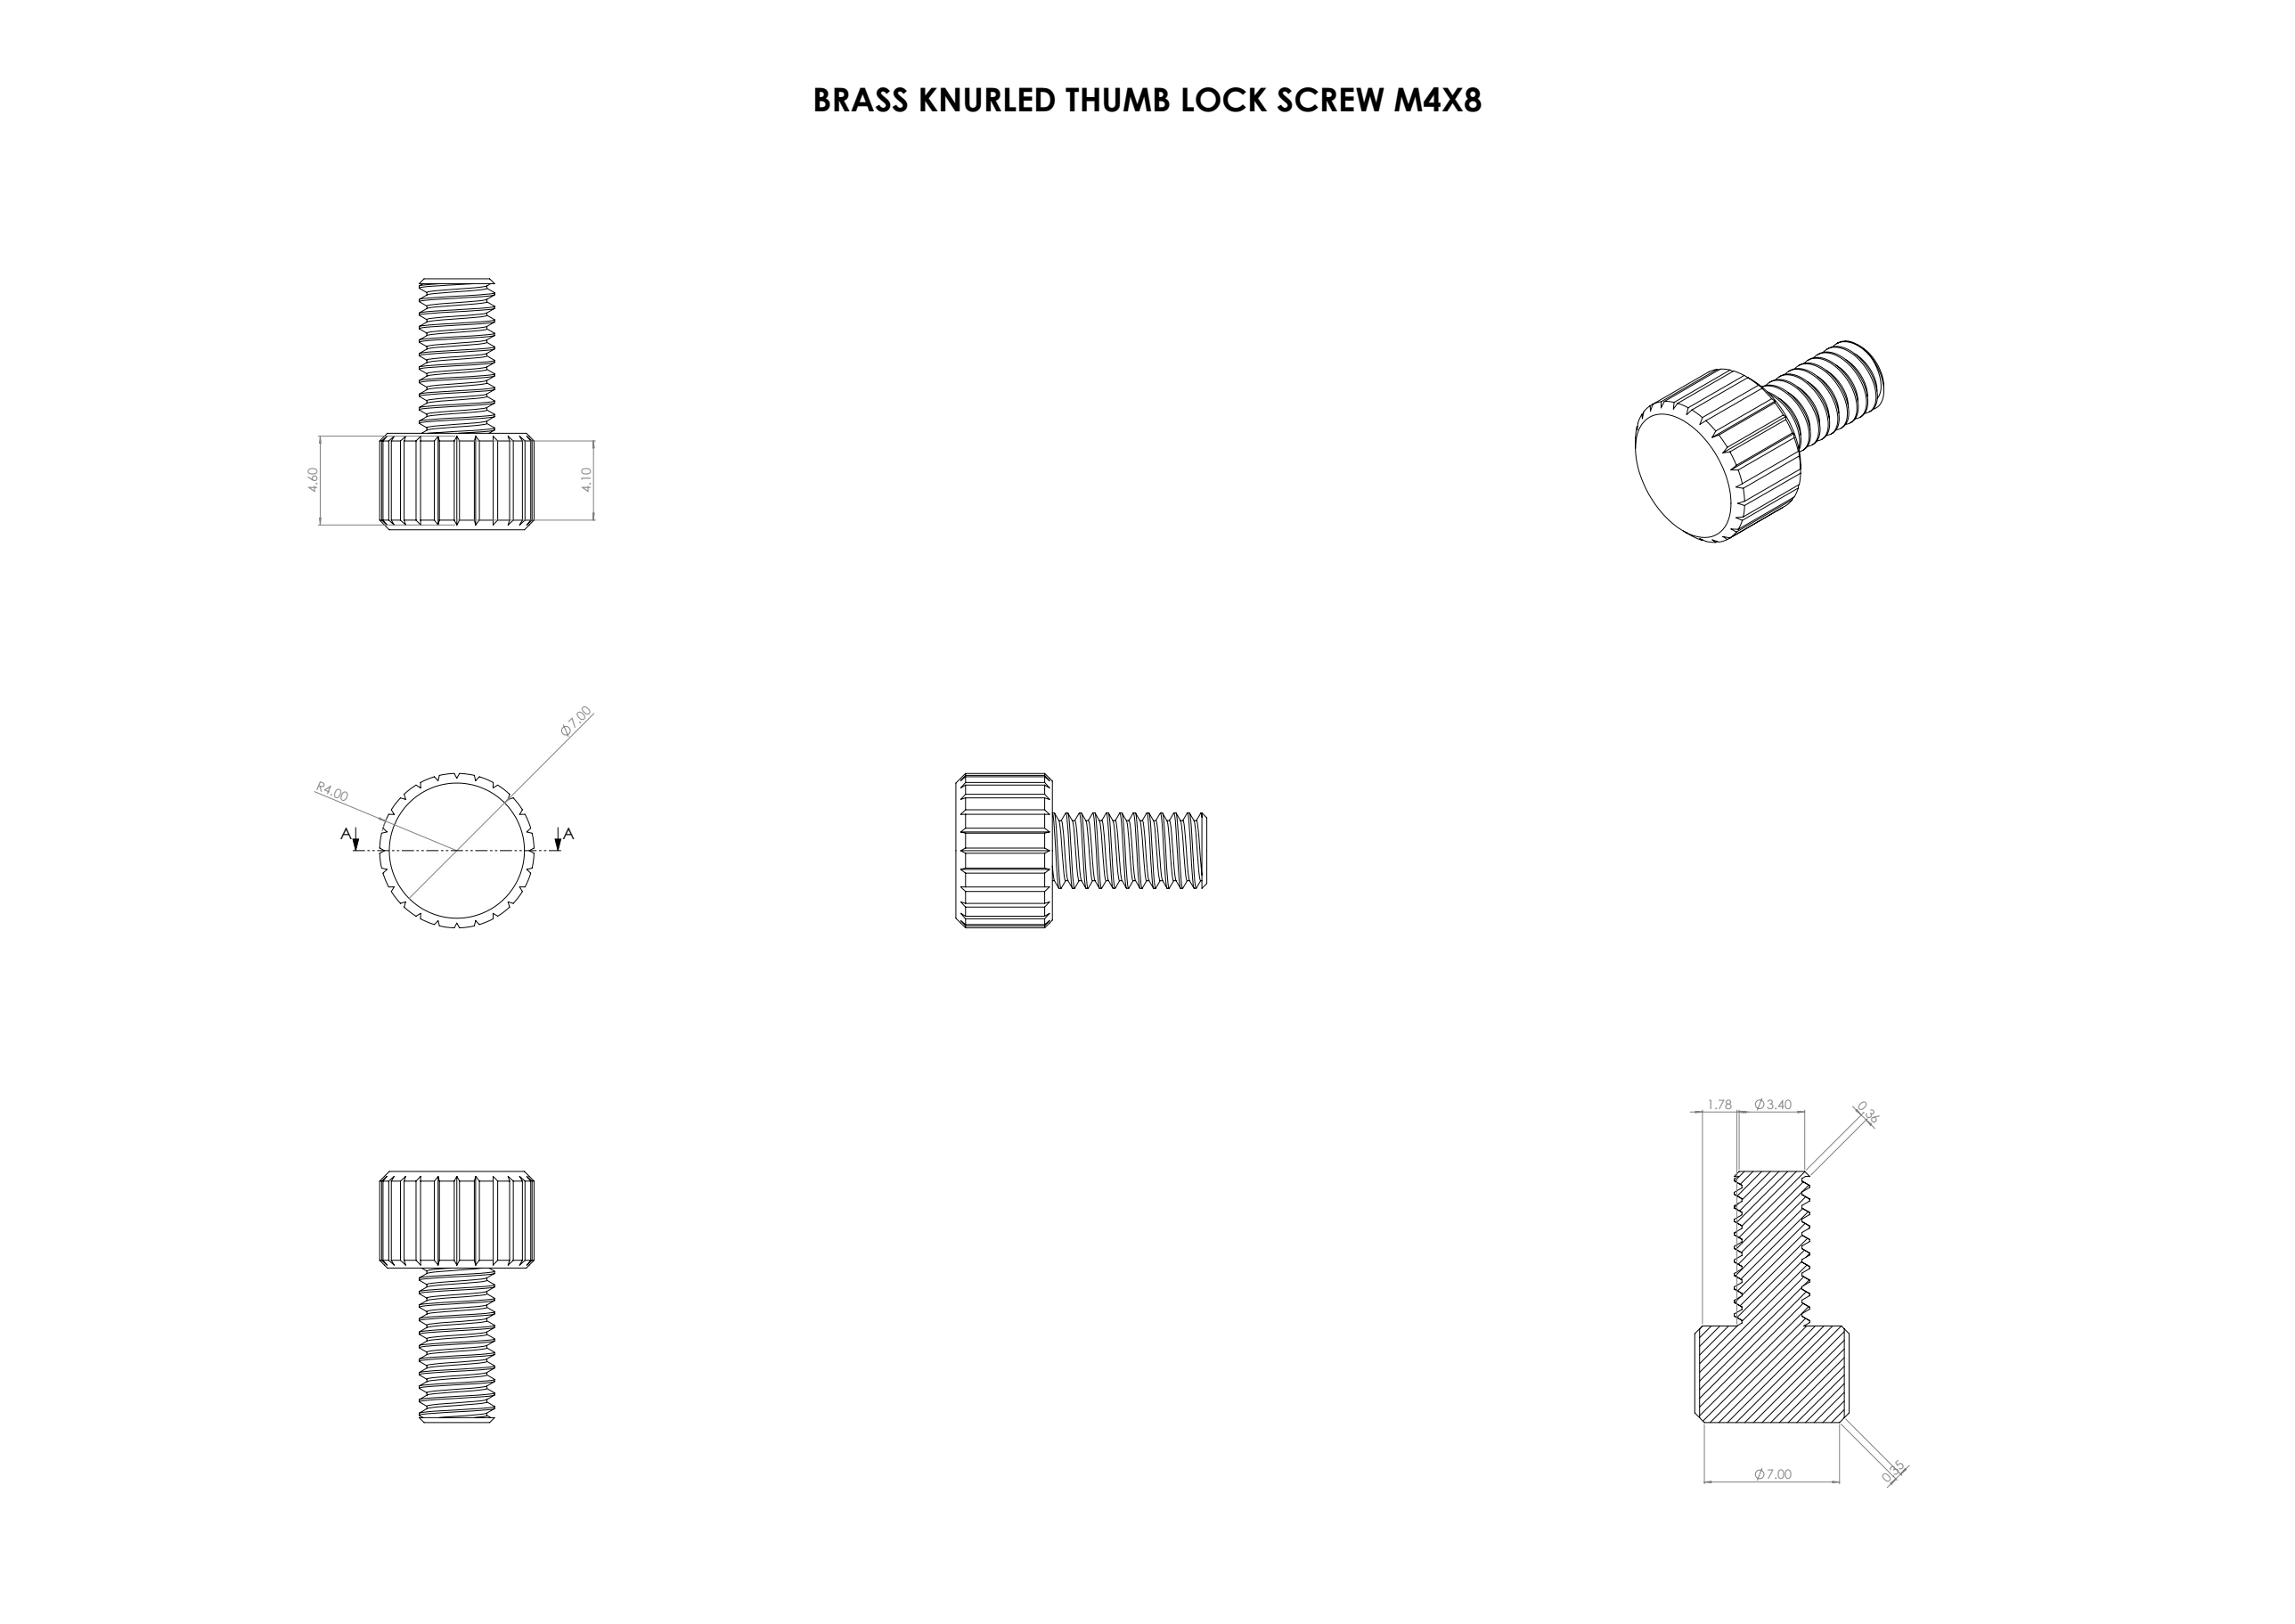
ISO-10303-21;
HEADER;
/* Generated by software containing ST-Developer
 * from STEP Tools, Inc. (www.steptools.com) 
 */

FILE_DESCRIPTION(
/* description */ (''),
/* implementation_level */ '2;1');

FILE_NAME(
/* name */ 
'12_Brass_Knurled_Thumb_Lock_Screw_M4x8.step',
/* time_stamp */ '2026-10-20T10:06:23-07:00',
/* author */ (''),
/* organization */ (''),
/* preprocessor_version */ 'ST-DEVELOPER v20.2',
/* originating_system */ 'Autodesk Translation Framework v15.15.0.0',
/* authorisation */ '');

FILE_SCHEMA (('AUTOMOTIVE_DESIGN { 1 0 10303 214 3 1 1 }'));
ENDSEC;

DATA;
#10=MECHANICAL_DESIGN_GEOMETRIC_PRESENTATION_REPRESENTATION('',(#473),#38611);
#336=(
BOUNDED_CURVE()
B_SPLINE_CURVE(2,(#37921,#37922,#37923),.UNSPECIFIED.,.F.,.F.)
B_SPLINE_CURVE_WITH_KNOTS((3,3),(0.0395243267589975,0.0757709160687003),
 .UNSPECIFIED.)
CURVE()
GEOMETRIC_REPRESENTATION_ITEM()
RATIONAL_B_SPLINE_CURVE((1.00144403367688,1.00138415709391,1.))
REPRESENTATION_ITEM('')
);
#337=(
BOUNDED_CURVE()
B_SPLINE_CURVE(2,(#37927,#37928,#37929),.UNSPECIFIED.,.F.,.F.)
B_SPLINE_CURVE_WITH_KNOTS((3,3),(0.,0.0368264807252771),.UNSPECIFIED.)
CURVE()
GEOMETRIC_REPRESENTATION_ITEM()
RATIONAL_B_SPLINE_CURVE((1.,1.00108727860041,1.00085032920655))
REPRESENTATION_ITEM('')
);
#338=(
BOUNDED_CURVE()
B_SPLINE_CURVE(2,(#37933,#37934,#37935),.UNSPECIFIED.,.F.,.F.)
B_SPLINE_CURVE_WITH_KNOTS((3,3),(0.,0.0362465893096916),.UNSPECIFIED.)
CURVE()
GEOMETRIC_REPRESENTATION_ITEM()
RATIONAL_B_SPLINE_CURVE((1.,1.00138415709372,1.00144403367668))
REPRESENTATION_ITEM('')
);
#339=(
BOUNDED_CURVE()
B_SPLINE_CURVE(2,(#37938,#37939,#37940),.UNSPECIFIED.,.F.,.F.)
B_SPLINE_CURVE_WITH_KNOTS((3,3),(0.023647462726297,0.0604739434515668),
 .UNSPECIFIED.)
CURVE()
GEOMETRIC_REPRESENTATION_ITEM()
RATIONAL_B_SPLINE_CURVE((1.00085032920655,1.0010872786004,1.))
REPRESENTATION_ITEM('')
);
#340=(
BOUNDED_CURVE()
B_SPLINE_CURVE(2,(#37944,#37945,#37946),.UNSPECIFIED.,.F.,.F.)
B_SPLINE_CURVE_WITH_KNOTS((3,3),(0.0395243267590134,0.0757709160687001),
 .UNSPECIFIED.)
CURVE()
GEOMETRIC_REPRESENTATION_ITEM()
RATIONAL_B_SPLINE_CURVE((1.00144403367689,1.00138415709393,1.))
REPRESENTATION_ITEM('')
);
#341=(
BOUNDED_CURVE()
B_SPLINE_CURVE(2,(#37950,#37951,#37952),.UNSPECIFIED.,.F.,.F.)
B_SPLINE_CURVE_WITH_KNOTS((3,3),(0.,0.036826480725251),.UNSPECIFIED.)
CURVE()
GEOMETRIC_REPRESENTATION_ITEM()
RATIONAL_B_SPLINE_CURVE((1.,1.00108727860024,1.00085032920643))
REPRESENTATION_ITEM('')
);
#342=(
BOUNDED_CURVE()
B_SPLINE_CURVE(2,(#37956,#37957,#37958),.UNSPECIFIED.,.F.,.F.)
B_SPLINE_CURVE_WITH_KNOTS((3,3),(0.,0.0362465893097029),.UNSPECIFIED.)
CURVE()
GEOMETRIC_REPRESENTATION_ITEM()
RATIONAL_B_SPLINE_CURVE((1.,1.00138415709418,1.00144403367715))
REPRESENTATION_ITEM('')
);
#343=(
BOUNDED_CURVE()
B_SPLINE_CURVE(2,(#37961,#37962,#37963),.UNSPECIFIED.,.F.,.F.)
B_SPLINE_CURVE_WITH_KNOTS((3,3),(0.0236474627262938,0.060473943451567),
 .UNSPECIFIED.)
CURVE()
GEOMETRIC_REPRESENTATION_ITEM()
RATIONAL_B_SPLINE_CURVE((1.00085032920586,1.00108727859952,1.))
REPRESENTATION_ITEM('')
);
#344=(
BOUNDED_CURVE()
B_SPLINE_CURVE(2,(#37967,#37968,#37969),.UNSPECIFIED.,.F.,.F.)
B_SPLINE_CURVE_WITH_KNOTS((3,3),(0.0395243267590093,0.0757709160687003),
 .UNSPECIFIED.)
CURVE()
GEOMETRIC_REPRESENTATION_ITEM()
RATIONAL_B_SPLINE_CURVE((1.00144403367677,1.00138415709381,1.))
REPRESENTATION_ITEM('')
);
#345=(
BOUNDED_CURVE()
B_SPLINE_CURVE(2,(#37973,#37974,#37975),.UNSPECIFIED.,.F.,.F.)
B_SPLINE_CURVE_WITH_KNOTS((3,3),(0.,0.0368264807252646),.UNSPECIFIED.)
CURVE()
GEOMETRIC_REPRESENTATION_ITEM()
RATIONAL_B_SPLINE_CURVE((1.,1.00108727859976,1.00085032920605))
REPRESENTATION_ITEM('')
);
#346=(
BOUNDED_CURVE()
B_SPLINE_CURVE(2,(#37979,#37980,#37981),.UNSPECIFIED.,.F.,.F.)
B_SPLINE_CURVE_WITH_KNOTS((3,3),(0.,0.0362465893097049),.UNSPECIFIED.)
CURVE()
GEOMETRIC_REPRESENTATION_ITEM()
RATIONAL_B_SPLINE_CURVE((1.,1.0013841570941,1.00144403367707))
REPRESENTATION_ITEM('')
);
#347=(
BOUNDED_CURVE()
B_SPLINE_CURVE(2,(#37984,#37985,#37986),.UNSPECIFIED.,.F.,.F.)
B_SPLINE_CURVE_WITH_KNOTS((3,3),(0.0236474627263067,0.0604739434515669),
 .UNSPECIFIED.)
CURVE()
GEOMETRIC_REPRESENTATION_ITEM()
RATIONAL_B_SPLINE_CURVE((1.00085032920563,1.00108727859922,1.))
REPRESENTATION_ITEM('')
);
#348=(
BOUNDED_CURVE()
B_SPLINE_CURVE(2,(#37990,#37991,#37992),.UNSPECIFIED.,.F.,.F.)
B_SPLINE_CURVE_WITH_KNOTS((3,3),(0.0395243267589975,0.0757709160687003),
 .UNSPECIFIED.)
CURVE()
GEOMETRIC_REPRESENTATION_ITEM()
RATIONAL_B_SPLINE_CURVE((1.00144403367688,1.00138415709391,1.))
REPRESENTATION_ITEM('')
);
#349=(
BOUNDED_CURVE()
B_SPLINE_CURVE(2,(#37996,#37997,#37998),.UNSPECIFIED.,.F.,.F.)
B_SPLINE_CURVE_WITH_KNOTS((3,3),(0.,0.0368264807252771),.UNSPECIFIED.)
CURVE()
GEOMETRIC_REPRESENTATION_ITEM()
RATIONAL_B_SPLINE_CURVE((1.,1.00108727860041,1.00085032920655))
REPRESENTATION_ITEM('')
);
#350=(
BOUNDED_CURVE()
B_SPLINE_CURVE(2,(#38002,#38003,#38004),.UNSPECIFIED.,.F.,.F.)
B_SPLINE_CURVE_WITH_KNOTS((3,3),(0.,0.0362465893096841),.UNSPECIFIED.)
CURVE()
GEOMETRIC_REPRESENTATION_ITEM()
RATIONAL_B_SPLINE_CURVE((1.,1.00138415709402,1.00144403367699))
REPRESENTATION_ITEM('')
);
#351=(
BOUNDED_CURVE()
B_SPLINE_CURVE(2,(#38007,#38008,#38009),.UNSPECIFIED.,.F.,.F.)
B_SPLINE_CURVE_WITH_KNOTS((3,3),(0.0236474627263223,0.0604739434515668),
 .UNSPECIFIED.)
CURVE()
GEOMETRIC_REPRESENTATION_ITEM()
RATIONAL_B_SPLINE_CURVE((1.00085032920605,1.00108727859975,1.))
REPRESENTATION_ITEM('')
);
#352=(
BOUNDED_CURVE()
B_SPLINE_CURVE(2,(#38013,#38014,#38015),.UNSPECIFIED.,.F.,.F.)
B_SPLINE_CURVE_WITH_KNOTS((3,3),(0.0395243267590166,0.0757709160687002),
 .UNSPECIFIED.)
CURVE()
GEOMETRIC_REPRESENTATION_ITEM()
RATIONAL_B_SPLINE_CURVE((1.00144403367685,1.00138415709388,1.))
REPRESENTATION_ITEM('')
);
#353=(
BOUNDED_CURVE()
B_SPLINE_CURVE(2,(#38019,#38020,#38021),.UNSPECIFIED.,.F.,.F.)
B_SPLINE_CURVE_WITH_KNOTS((3,3),(0.,0.0368264807252521),.UNSPECIFIED.)
CURVE()
GEOMETRIC_REPRESENTATION_ITEM()
RATIONAL_B_SPLINE_CURVE((1.,1.00108727859996,1.0008503292062))
REPRESENTATION_ITEM('')
);
#354=(
BOUNDED_CURVE()
B_SPLINE_CURVE(2,(#38025,#38026,#38027),.UNSPECIFIED.,.F.,.F.)
B_SPLINE_CURVE_WITH_KNOTS((3,3),(0.,0.0362465893096854),.UNSPECIFIED.)
CURVE()
GEOMETRIC_REPRESENTATION_ITEM()
RATIONAL_B_SPLINE_CURVE((1.,1.0013841570938,1.00144403367676))
REPRESENTATION_ITEM('')
);
#355=(
BOUNDED_CURVE()
B_SPLINE_CURVE(2,(#38030,#38031,#38032),.UNSPECIFIED.,.F.,.F.)
B_SPLINE_CURVE_WITH_KNOTS((3,3),(0.0236474627263314,0.0604739434515669),
 .UNSPECIFIED.)
CURVE()
GEOMETRIC_REPRESENTATION_ITEM()
RATIONAL_B_SPLINE_CURVE((1.00085032920606,1.00108727859977,1.))
REPRESENTATION_ITEM('')
);
#356=(
BOUNDED_CURVE()
B_SPLINE_CURVE(2,(#38036,#38037,#38038),.UNSPECIFIED.,.F.,.F.)
B_SPLINE_CURVE_WITH_KNOTS((3,3),(0.0395243267589997,0.0757709160687002),
 .UNSPECIFIED.)
CURVE()
GEOMETRIC_REPRESENTATION_ITEM()
RATIONAL_B_SPLINE_CURVE((1.00144403367698,1.00138415709401,1.))
REPRESENTATION_ITEM('')
);
#357=(
BOUNDED_CURVE()
B_SPLINE_CURVE(2,(#38042,#38043,#38044),.UNSPECIFIED.,.F.,.F.)
B_SPLINE_CURVE_WITH_KNOTS((3,3),(0.,0.0368264807252651),.UNSPECIFIED.)
CURVE()
GEOMETRIC_REPRESENTATION_ITEM()
RATIONAL_B_SPLINE_CURVE((1.,1.00108727860044,1.00085032920658))
REPRESENTATION_ITEM('')
);
#358=(
BOUNDED_CURVE()
B_SPLINE_CURVE(2,(#38048,#38049,#38050),.UNSPECIFIED.,.F.,.F.)
B_SPLINE_CURVE_WITH_KNOTS((3,3),(0.,0.0362465893096843),.UNSPECIFIED.)
CURVE()
GEOMETRIC_REPRESENTATION_ITEM()
RATIONAL_B_SPLINE_CURVE((1.,1.00138415709419,1.00144403367717))
REPRESENTATION_ITEM('')
);
#359=(
BOUNDED_CURVE()
B_SPLINE_CURVE(2,(#38053,#38054,#38055),.UNSPECIFIED.,.F.,.F.)
B_SPLINE_CURVE_WITH_KNOTS((3,3),(0.0236474627263023,0.060473943451567),
 .UNSPECIFIED.)
CURVE()
GEOMETRIC_REPRESENTATION_ITEM()
RATIONAL_B_SPLINE_CURVE((1.00085032920674,1.00108727860064,1.))
REPRESENTATION_ITEM('')
);
#360=(
BOUNDED_CURVE()
B_SPLINE_CURVE(2,(#38059,#38060,#38061),.UNSPECIFIED.,.F.,.F.)
B_SPLINE_CURVE_WITH_KNOTS((3,3),(0.0395243267590068,0.0757709160687003),
 .UNSPECIFIED.)
CURVE()
GEOMETRIC_REPRESENTATION_ITEM()
RATIONAL_B_SPLINE_CURVE((1.00144403367694,1.00138415709397,1.))
REPRESENTATION_ITEM('')
);
#361=(
BOUNDED_CURVE()
B_SPLINE_CURVE(2,(#38065,#38066,#38067),.UNSPECIFIED.,.F.,.F.)
B_SPLINE_CURVE_WITH_KNOTS((3,3),(0.,0.0368264807252612),.UNSPECIFIED.)
CURVE()
GEOMETRIC_REPRESENTATION_ITEM()
RATIONAL_B_SPLINE_CURVE((1.,1.00108727859988,1.00085032920614))
REPRESENTATION_ITEM('')
);
#362=(
BOUNDED_CURVE()
B_SPLINE_CURVE(2,(#38071,#38072,#38073),.UNSPECIFIED.,.F.,.F.)
B_SPLINE_CURVE_WITH_KNOTS((3,3),(0.,0.0362465893096925),.UNSPECIFIED.)
CURVE()
GEOMETRIC_REPRESENTATION_ITEM()
RATIONAL_B_SPLINE_CURVE((1.,1.00138415709391,1.00144403367687))
REPRESENTATION_ITEM('')
);
#363=(
BOUNDED_CURVE()
B_SPLINE_CURVE(2,(#38076,#38077,#38078),.UNSPECIFIED.,.F.,.F.)
B_SPLINE_CURVE_WITH_KNOTS((3,3),(0.0236474627263132,0.0604739434515669),
 .UNSPECIFIED.)
CURVE()
GEOMETRIC_REPRESENTATION_ITEM()
RATIONAL_B_SPLINE_CURVE((1.0008503292066,1.00108727860046,1.))
REPRESENTATION_ITEM('')
);
#364=(
BOUNDED_CURVE()
B_SPLINE_CURVE(2,(#38082,#38083,#38084),.UNSPECIFIED.,.F.,.F.)
B_SPLINE_CURVE_WITH_KNOTS((3,3),(0.039524326759018,0.0757709160687002),
 .UNSPECIFIED.)
CURVE()
GEOMETRIC_REPRESENTATION_ITEM()
RATIONAL_B_SPLINE_CURVE((1.00144403367702,1.00138415709405,1.))
REPRESENTATION_ITEM('')
);
#365=(
BOUNDED_CURVE()
B_SPLINE_CURVE(2,(#38088,#38089,#38090),.UNSPECIFIED.,.F.,.F.)
B_SPLINE_CURVE_WITH_KNOTS((3,3),(0.,0.0368264807252612),.UNSPECIFIED.)
CURVE()
GEOMETRIC_REPRESENTATION_ITEM()
RATIONAL_B_SPLINE_CURVE((1.,1.00108727860027,1.00085032920645))
REPRESENTATION_ITEM('')
);
#366=(
BOUNDED_CURVE()
B_SPLINE_CURVE(2,(#38094,#38095,#38096),.UNSPECIFIED.,.F.,.F.)
B_SPLINE_CURVE_WITH_KNOTS((3,3),(0.,0.0362465893096848),.UNSPECIFIED.)
CURVE()
GEOMETRIC_REPRESENTATION_ITEM()
RATIONAL_B_SPLINE_CURVE((1.,1.00138415709428,1.00144403367727))
REPRESENTATION_ITEM('')
);
#367=(
BOUNDED_CURVE()
B_SPLINE_CURVE(2,(#38099,#38100,#38101),.UNSPECIFIED.,.F.,.F.)
B_SPLINE_CURVE_WITH_KNOTS((3,3),(0.0236474627263229,0.060473943451567),
 .UNSPECIFIED.)
CURVE()
GEOMETRIC_REPRESENTATION_ITEM()
RATIONAL_B_SPLINE_CURVE((1.00085032920677,1.00108727860068,1.))
REPRESENTATION_ITEM('')
);
#368=(
BOUNDED_CURVE()
B_SPLINE_CURVE(2,(#38105,#38106,#38107),.UNSPECIFIED.,.F.,.F.)
B_SPLINE_CURVE_WITH_KNOTS((3,3),(0.0395243267590142,0.0757709160687002),
 .UNSPECIFIED.)
CURVE()
GEOMETRIC_REPRESENTATION_ITEM()
RATIONAL_B_SPLINE_CURVE((1.00144403367701,1.00138415709404,1.))
REPRESENTATION_ITEM('')
);
#369=(
BOUNDED_CURVE()
B_SPLINE_CURVE(2,(#38111,#38112,#38113),.UNSPECIFIED.,.F.,.F.)
B_SPLINE_CURVE_WITH_KNOTS((3,3),(0.,0.0368264807252614),.UNSPECIFIED.)
CURVE()
GEOMETRIC_REPRESENTATION_ITEM()
RATIONAL_B_SPLINE_CURVE((1.,1.00108727860056,1.00085032920667))
REPRESENTATION_ITEM('')
);
#370=(
BOUNDED_CURVE()
B_SPLINE_CURVE(2,(#38117,#38118,#38119),.UNSPECIFIED.,.F.,.F.)
B_SPLINE_CURVE_WITH_KNOTS((3,3),(0.,0.0362465893096775),.UNSPECIFIED.)
CURVE()
GEOMETRIC_REPRESENTATION_ITEM()
RATIONAL_B_SPLINE_CURVE((1.,1.00138415709412,1.0014440336771))
REPRESENTATION_ITEM('')
);
#371=(
BOUNDED_CURVE()
B_SPLINE_CURVE(2,(#38122,#38123,#38124),.UNSPECIFIED.,.F.,.F.)
B_SPLINE_CURVE_WITH_KNOTS((3,3),(0.023647462726333,0.060473943451567),
 .UNSPECIFIED.)
CURVE()
GEOMETRIC_REPRESENTATION_ITEM()
RATIONAL_B_SPLINE_CURVE((1.00085032920627,1.00108727860004,1.))
REPRESENTATION_ITEM('')
);
#372=(
BOUNDED_CURVE()
B_SPLINE_CURVE(2,(#38128,#38129,#38130),.UNSPECIFIED.,.F.,.F.)
B_SPLINE_CURVE_WITH_KNOTS((3,3),(0.0395243267590017,0.0757709160687002),
 .UNSPECIFIED.)
CURVE()
GEOMETRIC_REPRESENTATION_ITEM()
RATIONAL_B_SPLINE_CURVE((1.00144403367696,1.00138415709399,1.))
REPRESENTATION_ITEM('')
);
#373=(
BOUNDED_CURVE()
B_SPLINE_CURVE(2,(#38134,#38135,#38136),.UNSPECIFIED.,.F.,.F.)
B_SPLINE_CURVE_WITH_KNOTS((3,3),(0.,0.0368264807252428),.UNSPECIFIED.)
CURVE()
GEOMETRIC_REPRESENTATION_ITEM()
RATIONAL_B_SPLINE_CURVE((1.,1.00108727860007,1.0008503292063))
REPRESENTATION_ITEM('')
);
#374=(
BOUNDED_CURVE()
B_SPLINE_CURVE(2,(#38140,#38141,#38142),.UNSPECIFIED.,.F.,.F.)
B_SPLINE_CURVE_WITH_KNOTS((3,3),(0.,0.036246589309685),.UNSPECIFIED.)
CURVE()
GEOMETRIC_REPRESENTATION_ITEM()
RATIONAL_B_SPLINE_CURVE((1.,1.00138415709379,1.00144403367676))
REPRESENTATION_ITEM('')
);
#375=(
BOUNDED_CURVE()
B_SPLINE_CURVE(2,(#38145,#38146,#38147),.UNSPECIFIED.,.F.,.F.)
B_SPLINE_CURVE_WITH_KNOTS((3,3),(0.0236474627262961,0.060473943451567),
 .UNSPECIFIED.)
CURVE()
GEOMETRIC_REPRESENTATION_ITEM()
RATIONAL_B_SPLINE_CURVE((1.00085032920624,1.0010872786,1.))
REPRESENTATION_ITEM('')
);
#376=(
BOUNDED_CURVE()
B_SPLINE_CURVE(2,(#38151,#38152,#38153),.UNSPECIFIED.,.F.,.F.)
B_SPLINE_CURVE_WITH_KNOTS((3,3),(0.0395243267590158,0.0757709160687002),
 .UNSPECIFIED.)
CURVE()
GEOMETRIC_REPRESENTATION_ITEM()
RATIONAL_B_SPLINE_CURVE((1.0014440336769,1.00138415709393,1.))
REPRESENTATION_ITEM('')
);
#377=(
BOUNDED_CURVE()
B_SPLINE_CURVE(2,(#38157,#38158,#38159),.UNSPECIFIED.,.F.,.F.)
B_SPLINE_CURVE_WITH_KNOTS((3,3),(0.,0.0368264807252534),.UNSPECIFIED.)
CURVE()
GEOMETRIC_REPRESENTATION_ITEM()
RATIONAL_B_SPLINE_CURVE((1.,1.00108727860033,1.00085032920649))
REPRESENTATION_ITEM('')
);
#378=(
BOUNDED_CURVE()
B_SPLINE_CURVE(2,(#38163,#38164,#38165),.UNSPECIFIED.,.F.,.F.)
B_SPLINE_CURVE_WITH_KNOTS((3,3),(0.,0.0362465893096853),.UNSPECIFIED.)
CURVE()
GEOMETRIC_REPRESENTATION_ITEM()
RATIONAL_B_SPLINE_CURVE((1.,1.00138415709412,1.0014440336771))
REPRESENTATION_ITEM('')
);
#379=(
BOUNDED_CURVE()
B_SPLINE_CURVE(2,(#38168,#38169,#38170),.UNSPECIFIED.,.F.,.F.)
B_SPLINE_CURVE_WITH_KNOTS((3,3),(0.0236474627263147,0.060473943451567),
 .UNSPECIFIED.)
CURVE()
GEOMETRIC_REPRESENTATION_ITEM()
RATIONAL_B_SPLINE_CURVE((1.00085032920646,1.00108727860028,1.))
REPRESENTATION_ITEM('')
);
#380=(
BOUNDED_CURVE()
B_SPLINE_CURVE(2,(#38174,#38175,#38176),.UNSPECIFIED.,.F.,.F.)
B_SPLINE_CURVE_WITH_KNOTS((3,3),(0.0395243267590156,0.0757709160687002),
 .UNSPECIFIED.)
CURVE()
GEOMETRIC_REPRESENTATION_ITEM()
RATIONAL_B_SPLINE_CURVE((1.00144403367684,1.00138415709387,1.))
REPRESENTATION_ITEM('')
);
#381=(
BOUNDED_CURVE()
B_SPLINE_CURVE(2,(#38180,#38181,#38182),.UNSPECIFIED.,.F.,.F.)
B_SPLINE_CURVE_WITH_KNOTS((3,3),(0.,0.0368264807252693),.UNSPECIFIED.)
CURVE()
GEOMETRIC_REPRESENTATION_ITEM()
RATIONAL_B_SPLINE_CURVE((1.,1.00108727859986,1.00085032920613))
REPRESENTATION_ITEM('')
);
#382=(
BOUNDED_CURVE()
B_SPLINE_CURVE(2,(#38186,#38187,#38188),.UNSPECIFIED.,.F.,.F.)
B_SPLINE_CURVE_WITH_KNOTS((3,3),(0.,0.0362465893096901),.UNSPECIFIED.)
CURVE()
GEOMETRIC_REPRESENTATION_ITEM()
RATIONAL_B_SPLINE_CURVE((1.,1.00138415709395,1.00144403367692))
REPRESENTATION_ITEM('')
);
#383=(
BOUNDED_CURVE()
B_SPLINE_CURVE(2,(#38191,#38192,#38193),.UNSPECIFIED.,.F.,.F.)
B_SPLINE_CURVE_WITH_KNOTS((3,3),(0.0236474627263255,0.0604739434515669),
 .UNSPECIFIED.)
CURVE()
GEOMETRIC_REPRESENTATION_ITEM()
RATIONAL_B_SPLINE_CURVE((1.0008503292064,1.00108727860021,1.))
REPRESENTATION_ITEM('')
);
#384=(
BOUNDED_CURVE()
B_SPLINE_CURVE(2,(#38197,#38198,#38199),.UNSPECIFIED.,.F.,.F.)
B_SPLINE_CURVE_WITH_KNOTS((3,3),(0.0395243267590232,0.0757709160687003),
 .UNSPECIFIED.)
CURVE()
GEOMETRIC_REPRESENTATION_ITEM()
RATIONAL_B_SPLINE_CURVE((1.0014440336771,1.00138415709412,1.))
REPRESENTATION_ITEM('')
);
#385=(
BOUNDED_CURVE()
B_SPLINE_CURVE(2,(#38203,#38204,#38205),.UNSPECIFIED.,.F.,.F.)
B_SPLINE_CURVE_WITH_KNOTS((3,3),(0.,0.0368264807252497),.UNSPECIFIED.)
CURVE()
GEOMETRIC_REPRESENTATION_ITEM()
RATIONAL_B_SPLINE_CURVE((1.,1.00108727859942,1.00085032920579))
REPRESENTATION_ITEM('')
);
#386=(
BOUNDED_CURVE()
B_SPLINE_CURVE(2,(#38209,#38210,#38211),.UNSPECIFIED.,.F.,.F.)
B_SPLINE_CURVE_WITH_KNOTS((3,3),(0.,0.0362465893096849),.UNSPECIFIED.)
CURVE()
GEOMETRIC_REPRESENTATION_ITEM()
RATIONAL_B_SPLINE_CURVE((1.,1.00138415709363,1.00144403367659))
REPRESENTATION_ITEM('')
);
#387=(
BOUNDED_CURVE()
B_SPLINE_CURVE(2,(#38214,#38215,#38216),.UNSPECIFIED.,.F.,.F.)
B_SPLINE_CURVE_WITH_KNOTS((3,3),(0.0236474627263162,0.060473943451567),
 .UNSPECIFIED.)
CURVE()
GEOMETRIC_REPRESENTATION_ITEM()
RATIONAL_B_SPLINE_CURVE((1.00085032920633,1.00108727860012,1.))
REPRESENTATION_ITEM('')
);
#388=(
BOUNDED_CURVE()
B_SPLINE_CURVE(2,(#38220,#38221,#38222),.UNSPECIFIED.,.F.,.F.)
B_SPLINE_CURVE_WITH_KNOTS((3,3),(0.0395243267590082,0.0757709160687002),
 .UNSPECIFIED.)
CURVE()
GEOMETRIC_REPRESENTATION_ITEM()
RATIONAL_B_SPLINE_CURVE((1.00144403367716,1.00138415709418,1.))
REPRESENTATION_ITEM('')
);
#389=(
BOUNDED_CURVE()
B_SPLINE_CURVE(2,(#38226,#38227,#38228),.UNSPECIFIED.,.F.,.F.)
B_SPLINE_CURVE_WITH_KNOTS((3,3),(0.,0.0368264807252609),.UNSPECIFIED.)
CURVE()
GEOMETRIC_REPRESENTATION_ITEM()
RATIONAL_B_SPLINE_CURVE((1.,1.00108727859987,1.00085032920614))
REPRESENTATION_ITEM('')
);
#390=(
BOUNDED_CURVE()
B_SPLINE_CURVE(2,(#38232,#38233,#38234),.UNSPECIFIED.,.F.,.F.)
B_SPLINE_CURVE_WITH_KNOTS((3,3),(0.,0.0362465893096812),.UNSPECIFIED.)
CURVE()
GEOMETRIC_REPRESENTATION_ITEM()
RATIONAL_B_SPLINE_CURVE((1.,1.0013841570937,1.00144403367666))
REPRESENTATION_ITEM('')
);
#391=(
BOUNDED_CURVE()
B_SPLINE_CURVE(2,(#38237,#38238,#38239),.UNSPECIFIED.,.F.,.F.)
B_SPLINE_CURVE_WITH_KNOTS((3,3),(0.0236474627263107,0.0604739434515669),
 .UNSPECIFIED.)
CURVE()
GEOMETRIC_REPRESENTATION_ITEM()
RATIONAL_B_SPLINE_CURVE((1.00085032920669,1.00108727860058,1.))
REPRESENTATION_ITEM('')
);
#392=(
BOUNDED_CURVE()
B_SPLINE_CURVE(2,(#38243,#38244,#38245),.UNSPECIFIED.,.F.,.F.)
B_SPLINE_CURVE_WITH_KNOTS((3,3),(0.0395243267589996,0.0757709160687002),
 .UNSPECIFIED.)
CURVE()
GEOMETRIC_REPRESENTATION_ITEM()
RATIONAL_B_SPLINE_CURVE((1.00144403367705,1.00138415709408,1.))
REPRESENTATION_ITEM('')
);
#393=(
BOUNDED_CURVE()
B_SPLINE_CURVE(2,(#38249,#38250,#38251),.UNSPECIFIED.,.F.,.F.)
B_SPLINE_CURVE_WITH_KNOTS((3,3),(0.,0.0368264807252541),.UNSPECIFIED.)
CURVE()
GEOMETRIC_REPRESENTATION_ITEM()
RATIONAL_B_SPLINE_CURVE((1.,1.00108727860017,1.00085032920637))
REPRESENTATION_ITEM('')
);
#394=(
BOUNDED_CURVE()
B_SPLINE_CURVE(2,(#38255,#38256,#38257),.UNSPECIFIED.,.F.,.F.)
B_SPLINE_CURVE_WITH_KNOTS((3,3),(0.,0.0362465893096801),.UNSPECIFIED.)
CURVE()
GEOMETRIC_REPRESENTATION_ITEM()
RATIONAL_B_SPLINE_CURVE((1.,1.00138415709414,1.00144403367712))
REPRESENTATION_ITEM('')
);
#395=(
BOUNDED_CURVE()
B_SPLINE_CURVE(2,(#38260,#38261,#38262),.UNSPECIFIED.,.F.,.F.)
B_SPLINE_CURVE_WITH_KNOTS((3,3),(0.0236474627263037,0.060473943451567),
 .UNSPECIFIED.)
CURVE()
GEOMETRIC_REPRESENTATION_ITEM()
RATIONAL_B_SPLINE_CURVE((1.00085032920654,1.00108727860038,1.))
REPRESENTATION_ITEM('')
);
#396=(
BOUNDED_CURVE()
B_SPLINE_CURVE(2,(#38266,#38267,#38268),.UNSPECIFIED.,.F.,.F.)
B_SPLINE_CURVE_WITH_KNOTS((3,3),(0.0395243267590246,0.0757709160687002),
 .UNSPECIFIED.)
CURVE()
GEOMETRIC_REPRESENTATION_ITEM()
RATIONAL_B_SPLINE_CURVE((1.00144403367709,1.00138415709411,1.))
REPRESENTATION_ITEM('')
);
#397=(
BOUNDED_CURVE()
B_SPLINE_CURVE(2,(#38272,#38273,#38274),.UNSPECIFIED.,.F.,.F.)
B_SPLINE_CURVE_WITH_KNOTS((3,3),(0.,0.0368264807252722),.UNSPECIFIED.)
CURVE()
GEOMETRIC_REPRESENTATION_ITEM()
RATIONAL_B_SPLINE_CURVE((1.,1.00108727859999,1.00085032920623))
REPRESENTATION_ITEM('')
);
#398=(
BOUNDED_CURVE()
B_SPLINE_CURVE(2,(#38278,#38279,#38280),.UNSPECIFIED.,.F.,.F.)
B_SPLINE_CURVE_WITH_KNOTS((3,3),(0.,0.036246589309683),.UNSPECIFIED.)
CURVE()
GEOMETRIC_REPRESENTATION_ITEM()
RATIONAL_B_SPLINE_CURVE((1.,1.00138415709414,1.00144403367712))
REPRESENTATION_ITEM('')
);
#399=(
BOUNDED_CURVE()
B_SPLINE_CURVE(2,(#38283,#38284,#38285),.UNSPECIFIED.,.F.,.F.)
B_SPLINE_CURVE_WITH_KNOTS((3,3),(0.0236474627263149,0.060473943451567),
 .UNSPECIFIED.)
CURVE()
GEOMETRIC_REPRESENTATION_ITEM()
RATIONAL_B_SPLINE_CURVE((1.00085032920643,1.00108727860025,1.))
REPRESENTATION_ITEM('')
);
#400=(
BOUNDED_CURVE()
B_SPLINE_CURVE(2,(#38289,#38290,#38291),.UNSPECIFIED.,.F.,.F.)
B_SPLINE_CURVE_WITH_KNOTS((3,3),(0.0395243267590166,0.0757709160687002),
 .UNSPECIFIED.)
CURVE()
GEOMETRIC_REPRESENTATION_ITEM()
RATIONAL_B_SPLINE_CURVE((1.00144403367727,1.00138415709429,1.))
REPRESENTATION_ITEM('')
);
#401=(
BOUNDED_CURVE()
B_SPLINE_CURVE(2,(#38295,#38296,#38297),.UNSPECIFIED.,.F.,.F.)
B_SPLINE_CURVE_WITH_KNOTS((3,3),(0.,0.0368264807252481),.UNSPECIFIED.)
CURVE()
GEOMETRIC_REPRESENTATION_ITEM()
RATIONAL_B_SPLINE_CURVE((1.,1.00108727859946,1.00085032920581))
REPRESENTATION_ITEM('')
);
#402=(
BOUNDED_CURVE()
B_SPLINE_CURVE(2,(#38301,#38302,#38303),.UNSPECIFIED.,.F.,.F.)
B_SPLINE_CURVE_WITH_KNOTS((3,3),(0.,0.0362465893096797),.UNSPECIFIED.)
CURVE()
GEOMETRIC_REPRESENTATION_ITEM()
RATIONAL_B_SPLINE_CURVE((1.,1.00138415709394,1.00144403367691))
REPRESENTATION_ITEM('')
);
#403=(
BOUNDED_CURVE()
B_SPLINE_CURVE(2,(#38306,#38307,#38308),.UNSPECIFIED.,.F.,.F.)
B_SPLINE_CURVE_WITH_KNOTS((3,3),(0.0236474627263141,0.0604739434515669),
 .UNSPECIFIED.)
CURVE()
GEOMETRIC_REPRESENTATION_ITEM()
RATIONAL_B_SPLINE_CURVE((1.00085032920622,1.00108727859997,1.))
REPRESENTATION_ITEM('')
);
#404=(
BOUNDED_CURVE()
B_SPLINE_CURVE(2,(#38312,#38313,#38314),.UNSPECIFIED.,.F.,.F.)
B_SPLINE_CURVE_WITH_KNOTS((3,3),(0.0395243267590075,0.0757709160687003),
 .UNSPECIFIED.)
CURVE()
GEOMETRIC_REPRESENTATION_ITEM()
RATIONAL_B_SPLINE_CURVE((1.00144403367703,1.00138415709406,1.))
REPRESENTATION_ITEM('')
);
#405=(
BOUNDED_CURVE()
B_SPLINE_CURVE(2,(#38318,#38319,#38320),.UNSPECIFIED.,.F.,.F.)
B_SPLINE_CURVE_WITH_KNOTS((3,3),(0.,0.0368264807252487),.UNSPECIFIED.)
CURVE()
GEOMETRIC_REPRESENTATION_ITEM()
RATIONAL_B_SPLINE_CURVE((1.,1.00108727859994,1.00085032920619))
REPRESENTATION_ITEM('')
);
#406=(
BOUNDED_CURVE()
B_SPLINE_CURVE(2,(#38324,#38325,#38326),.UNSPECIFIED.,.F.,.F.)
B_SPLINE_CURVE_WITH_KNOTS((3,3),(0.,0.0362465893096912),.UNSPECIFIED.)
CURVE()
GEOMETRIC_REPRESENTATION_ITEM()
RATIONAL_B_SPLINE_CURVE((1.,1.00138415709428,1.00144403367727))
REPRESENTATION_ITEM('')
);
#407=(
BOUNDED_CURVE()
B_SPLINE_CURVE(2,(#38329,#38330,#38331),.UNSPECIFIED.,.F.,.F.)
B_SPLINE_CURVE_WITH_KNOTS((3,3),(0.0236474627263162,0.0604739434515669),
 .UNSPECIFIED.)
CURVE()
GEOMETRIC_REPRESENTATION_ITEM()
RATIONAL_B_SPLINE_CURVE((1.00085032920654,1.00108727860038,1.))
REPRESENTATION_ITEM('')
);
#408=(
BOUNDED_CURVE()
B_SPLINE_CURVE(2,(#38335,#38336,#38337),.UNSPECIFIED.,.F.,.F.)
B_SPLINE_CURVE_WITH_KNOTS((3,3),(0.0395243267590164,0.0757709160687002),
 .UNSPECIFIED.)
CURVE()
GEOMETRIC_REPRESENTATION_ITEM()
RATIONAL_B_SPLINE_CURVE((1.0014440336769,1.00138415709393,1.))
REPRESENTATION_ITEM('')
);
#409=(
BOUNDED_CURVE()
B_SPLINE_CURVE(2,(#38341,#38342,#38343),.UNSPECIFIED.,.F.,.F.)
B_SPLINE_CURVE_WITH_KNOTS((3,3),(0.,0.0368264807252535),.UNSPECIFIED.)
CURVE()
GEOMETRIC_REPRESENTATION_ITEM()
RATIONAL_B_SPLINE_CURVE((1.,1.00108727860031,1.00085032920648))
REPRESENTATION_ITEM('')
);
#410=(
BOUNDED_CURVE()
B_SPLINE_CURVE(2,(#38347,#38348,#38349),.UNSPECIFIED.,.F.,.F.)
B_SPLINE_CURVE_WITH_KNOTS((3,3),(0.,0.0362465893096775),.UNSPECIFIED.)
CURVE()
GEOMETRIC_REPRESENTATION_ITEM()
RATIONAL_B_SPLINE_CURVE((1.,1.00138415709412,1.0014440336771))
REPRESENTATION_ITEM('')
);
#411=(
BOUNDED_CURVE()
B_SPLINE_CURVE(2,(#38352,#38353,#38354),.UNSPECIFIED.,.F.,.F.)
B_SPLINE_CURVE_WITH_KNOTS((3,3),(0.023647462726333,0.060473943451567),
 .UNSPECIFIED.)
CURVE()
GEOMETRIC_REPRESENTATION_ITEM()
RATIONAL_B_SPLINE_CURVE((1.00085032920627,1.00108727860004,1.))
REPRESENTATION_ITEM('')
);
#412=(
BOUNDED_CURVE()
B_SPLINE_CURVE(2,(#38358,#38359,#38360),.UNSPECIFIED.,.F.,.F.)
B_SPLINE_CURVE_WITH_KNOTS((3,3),(0.03952432675902,0.0757709160687003),
 .UNSPECIFIED.)
CURVE()
GEOMETRIC_REPRESENTATION_ITEM()
RATIONAL_B_SPLINE_CURVE((1.00144403367664,1.00138415709369,1.))
REPRESENTATION_ITEM('')
);
#413=(
BOUNDED_CURVE()
B_SPLINE_CURVE(2,(#38364,#38365,#38366),.UNSPECIFIED.,.F.,.F.)
B_SPLINE_CURVE_WITH_KNOTS((3,3),(0.,0.0368264807252641),.UNSPECIFIED.)
CURVE()
GEOMETRIC_REPRESENTATION_ITEM()
RATIONAL_B_SPLINE_CURVE((1.,1.00108727860008,1.0008503292063))
REPRESENTATION_ITEM('')
);
#414=(
BOUNDED_CURVE()
B_SPLINE_CURVE(2,(#38370,#38371,#38372),.UNSPECIFIED.,.F.,.F.)
B_SPLINE_CURVE_WITH_KNOTS((3,3),(0.,0.0362465893096867),.UNSPECIFIED.)
CURVE()
GEOMETRIC_REPRESENTATION_ITEM()
RATIONAL_B_SPLINE_CURVE((1.,1.00138415709384,1.0014440336768))
REPRESENTATION_ITEM('')
);
#415=(
BOUNDED_CURVE()
B_SPLINE_CURVE(2,(#38375,#38376,#38377),.UNSPECIFIED.,.F.,.F.)
B_SPLINE_CURVE_WITH_KNOTS((3,3),(0.0236474627263162,0.060473943451567),
 .UNSPECIFIED.)
CURVE()
GEOMETRIC_REPRESENTATION_ITEM()
RATIONAL_B_SPLINE_CURVE((1.00085032920569,1.0010872785993,1.))
REPRESENTATION_ITEM('')
);
#416=(
BOUNDED_CURVE()
B_SPLINE_CURVE(2,(#38381,#38382,#38383),.UNSPECIFIED.,.F.,.F.)
B_SPLINE_CURVE_WITH_KNOTS((3,3),(0.0395243267590018,0.0757709160687002),
 .UNSPECIFIED.)
CURVE()
GEOMETRIC_REPRESENTATION_ITEM()
RATIONAL_B_SPLINE_CURVE((1.00144403367701,1.00138415709404,1.))
REPRESENTATION_ITEM('')
);
#417=(
BOUNDED_CURVE()
B_SPLINE_CURVE(2,(#38387,#38388,#38389),.UNSPECIFIED.,.F.,.F.)
B_SPLINE_CURVE_WITH_KNOTS((3,3),(0.,0.0368264807252595),.UNSPECIFIED.)
CURVE()
GEOMETRIC_REPRESENTATION_ITEM()
RATIONAL_B_SPLINE_CURVE((1.,1.00108727860035,1.00085032920651))
REPRESENTATION_ITEM('')
);
#418=(
BOUNDED_CURVE()
B_SPLINE_CURVE(2,(#38393,#38394,#38395),.UNSPECIFIED.,.F.,.F.)
B_SPLINE_CURVE_WITH_KNOTS((3,3),(0.,0.0362465893096985),.UNSPECIFIED.)
CURVE()
GEOMETRIC_REPRESENTATION_ITEM()
RATIONAL_B_SPLINE_CURVE((1.,1.00138415709386,1.00144403367682))
REPRESENTATION_ITEM('')
);
#419=(
BOUNDED_CURVE()
B_SPLINE_CURVE(2,(#38398,#38399,#38400),.UNSPECIFIED.,.F.,.F.)
B_SPLINE_CURVE_WITH_KNOTS((3,3),(0.0236474627262938,0.060473943451567),
 .UNSPECIFIED.)
CURVE()
GEOMETRIC_REPRESENTATION_ITEM()
RATIONAL_B_SPLINE_CURVE((1.00085032920587,1.00108727859953,1.))
REPRESENTATION_ITEM('')
);
#420=(
BOUNDED_CURVE()
B_SPLINE_CURVE(2,(#38404,#38405,#38406),.UNSPECIFIED.,.F.,.F.)
B_SPLINE_CURVE_WITH_KNOTS((3,3),(0.0395243267590063,0.0757709160687004),
 .UNSPECIFIED.)
CURVE()
GEOMETRIC_REPRESENTATION_ITEM()
RATIONAL_B_SPLINE_CURVE((1.00144403367682,1.00138415709386,1.))
REPRESENTATION_ITEM('')
);
#421=(
BOUNDED_CURVE()
B_SPLINE_CURVE(2,(#38410,#38411,#38412),.UNSPECIFIED.,.F.,.F.)
B_SPLINE_CURVE_WITH_KNOTS((3,3),(0.,0.0368264807252569),.UNSPECIFIED.)
CURVE()
GEOMETRIC_REPRESENTATION_ITEM()
RATIONAL_B_SPLINE_CURVE((1.,1.00108727859996,1.00085032920621))
REPRESENTATION_ITEM('')
);
#422=(
BOUNDED_CURVE()
B_SPLINE_CURVE(2,(#38416,#38417,#38418),.UNSPECIFIED.,.F.,.F.)
B_SPLINE_CURVE_WITH_KNOTS((3,3),(0.,0.0362465893096971),.UNSPECIFIED.)
CURVE()
GEOMETRIC_REPRESENTATION_ITEM()
RATIONAL_B_SPLINE_CURVE((1.,1.00138415709408,1.00144403367705))
REPRESENTATION_ITEM('')
);
#423=(
BOUNDED_CURVE()
B_SPLINE_CURVE(2,(#38421,#38422,#38423),.UNSPECIFIED.,.F.,.F.)
B_SPLINE_CURVE_WITH_KNOTS((3,3),(0.0236474627263185,0.0604739434515669),
 .UNSPECIFIED.)
CURVE()
GEOMETRIC_REPRESENTATION_ITEM()
RATIONAL_B_SPLINE_CURVE((1.00085032920632,1.0010872786001,1.))
REPRESENTATION_ITEM('')
);
#424=(
BOUNDED_CURVE()
B_SPLINE_CURVE(2,(#38427,#38428,#38429),.UNSPECIFIED.,.F.,.F.)
B_SPLINE_CURVE_WITH_KNOTS((3,3),(0.0395243267590211,0.0757709160687003),
 .UNSPECIFIED.)
CURVE()
GEOMETRIC_REPRESENTATION_ITEM()
RATIONAL_B_SPLINE_CURVE((1.00144403367694,1.00138415709397,1.))
REPRESENTATION_ITEM('')
);
#425=(
BOUNDED_CURVE()
B_SPLINE_CURVE(2,(#38433,#38434,#38435),.UNSPECIFIED.,.F.,.F.)
B_SPLINE_CURVE_WITH_KNOTS((3,3),(0.,0.0368264807252641),.UNSPECIFIED.)
CURVE()
GEOMETRIC_REPRESENTATION_ITEM()
RATIONAL_B_SPLINE_CURVE((1.,1.00108727860008,1.0008503292063))
REPRESENTATION_ITEM('')
);
#426=(
BOUNDED_CURVE()
B_SPLINE_CURVE(2,(#38439,#38440,#38441),.UNSPECIFIED.,.F.,.F.)
B_SPLINE_CURVE_WITH_KNOTS((3,3),(0.,0.0362465893097037),.UNSPECIFIED.)
CURVE()
GEOMETRIC_REPRESENTATION_ITEM()
RATIONAL_B_SPLINE_CURVE((1.,1.00138415709397,1.00144403367693))
REPRESENTATION_ITEM('')
);
#427=(
BOUNDED_CURVE()
B_SPLINE_CURVE(2,(#38444,#38445,#38446),.UNSPECIFIED.,.F.,.F.)
B_SPLINE_CURVE_WITH_KNOTS((3,3),(0.023647462726311,0.0604739434515669),
 .UNSPECIFIED.)
CURVE()
GEOMETRIC_REPRESENTATION_ITEM()
RATIONAL_B_SPLINE_CURVE((1.00085032920618,1.00108727859993,1.))
REPRESENTATION_ITEM('')
);
#428=(
BOUNDED_CURVE()
B_SPLINE_CURVE(2,(#38450,#38451,#38452),.UNSPECIFIED.,.F.,.F.)
B_SPLINE_CURVE_WITH_KNOTS((3,3),(0.0395243267590132,0.0757709160687002),
 .UNSPECIFIED.)
CURVE()
GEOMETRIC_REPRESENTATION_ITEM()
RATIONAL_B_SPLINE_CURVE((1.00144403367714,1.00138415709416,1.))
REPRESENTATION_ITEM('')
);
#429=(
BOUNDED_CURVE()
B_SPLINE_CURVE(2,(#38456,#38457,#38458),.UNSPECIFIED.,.F.,.F.)
B_SPLINE_CURVE_WITH_KNOTS((3,3),(0.,0.0368264807252791),.UNSPECIFIED.)
CURVE()
GEOMETRIC_REPRESENTATION_ITEM()
RATIONAL_B_SPLINE_CURVE((1.,1.0010872786001,1.00085032920631))
REPRESENTATION_ITEM('')
);
#430=(
BOUNDED_CURVE()
B_SPLINE_CURVE(2,(#38462,#38463,#38464),.UNSPECIFIED.,.F.,.F.)
B_SPLINE_CURVE_WITH_KNOTS((3,3),(0.,0.0362465893096923),.UNSPECIFIED.)
CURVE()
GEOMETRIC_REPRESENTATION_ITEM()
RATIONAL_B_SPLINE_CURVE((1.,1.00138415709398,1.00144403367695))
REPRESENTATION_ITEM('')
);
#431=(
BOUNDED_CURVE()
B_SPLINE_CURVE(2,(#38467,#38468,#38469),.UNSPECIFIED.,.F.,.F.)
B_SPLINE_CURVE_WITH_KNOTS((3,3),(0.0236474627263034,0.060473943451567),
 .UNSPECIFIED.)
CURVE()
GEOMETRIC_REPRESENTATION_ITEM()
RATIONAL_B_SPLINE_CURVE((1.00085032920706,1.00108727860106,1.))
REPRESENTATION_ITEM('')
);
#445=SHAPE_REPRESENTATION_RELATIONSHIP('SRR','None',#38681,#459);
#459=ADVANCED_BREP_SHAPE_REPRESENTATION('',(#487),#38610);
#473=STYLED_ITEM('',(#38885),#487);
#487=MANIFOLD_SOLID_BREP('Thumb screw',#16247);
#508=B_SPLINE_SURFACE_WITH_KNOTS('',3,3,((#37042,#37043,#37044,#37045,#37046,
#37047,#37048,#37049,#37050,#37051,#37052,#37053,#37054,#37055,#37056,#37057,
#37058,#37059,#37060,#37061,#37062,#37063,#37064,#37065,#37066,#37067,#37068,
#37069,#37070,#37071,#37072,#37073,#37074,#37075,#37076,#37077,#37078,#37079,
#37080,#37081,#37082,#37083,#37084,#37085,#37086,#37087,#37088,#37089,#37090,
#37091,#37092,#37093,#37094,#37095,#37096,#37097,#37098,#37099,#37100,#37101,
#37102,#37103,#37104,#37105,#37106,#37107,#37108,#37109,#37110,#37111,#37112,
#37113,#37114,#37115,#37116),(#37117,#37118,#37119,#37120,#37121,#37122,
#37123,#37124,#37125,#37126,#37127,#37128,#37129,#37130,#37131,#37132,#37133,
#37134,#37135,#37136,#37137,#37138,#37139,#37140,#37141,#37142,#37143,#37144,
#37145,#37146,#37147,#37148,#37149,#37150,#37151,#37152,#37153,#37154,#37155,
#37156,#37157,#37158,#37159,#37160,#37161,#37162,#37163,#37164,#37165,#37166,
#37167,#37168,#37169,#37170,#37171,#37172,#37173,#37174,#37175,#37176,#37177,
#37178,#37179,#37180,#37181,#37182,#37183,#37184,#37185,#37186,#37187,#37188,
#37189,#37190,#37191),(#37192,#37193,#37194,#37195,#37196,#37197,#37198,
#37199,#37200,#37201,#37202,#37203,#37204,#37205,#37206,#37207,#37208,#37209,
#37210,#37211,#37212,#37213,#37214,#37215,#37216,#37217,#37218,#37219,#37220,
#37221,#37222,#37223,#37224,#37225,#37226,#37227,#37228,#37229,#37230,#37231,
#37232,#37233,#37234,#37235,#37236,#37237,#37238,#37239,#37240,#37241,#37242,
#37243,#37244,#37245,#37246,#37247,#37248,#37249,#37250,#37251,#37252,#37253,
#37254,#37255,#37256,#37257,#37258,#37259,#37260,#37261,#37262,#37263,#37264,
#37265,#37266),(#37267,#37268,#37269,#37270,#37271,#37272,#37273,#37274,
#37275,#37276,#37277,#37278,#37279,#37280,#37281,#37282,#37283,#37284,#37285,
#37286,#37287,#37288,#37289,#37290,#37291,#37292,#37293,#37294,#37295,#37296,
#37297,#37298,#37299,#37300,#37301,#37302,#37303,#37304,#37305,#37306,#37307,
#37308,#37309,#37310,#37311,#37312,#37313,#37314,#37315,#37316,#37317,#37318,
#37319,#37320,#37321,#37322,#37323,#37324,#37325,#37326,#37327,#37328,#37329,
#37330,#37331,#37332,#37333,#37334,#37335,#37336,#37337,#37338,#37339,#37340,
#37341)),.UNSPECIFIED.,.F.,.F.,.F.,(4,4),(4,1,1,1,1,1,1,1,1,1,1,1,1,1,1,
1,1,1,1,1,1,1,1,1,1,1,1,1,1,1,1,1,1,1,1,1,1,1,1,1,1,1,1,1,1,1,1,1,1,1,1,
1,1,1,1,1,1,1,1,1,1,1,1,1,1,1,1,1,1,1,1,1,4),(0.,0.0460148164544132),(8.31058692273973,
9.30493516644425,10.2992834101488,11.2936316538533,12.2879798975578,13.2823281412623,
14.2766763849668,15.2710246286714,16.2653728723759,17.2597211160804,18.2540693597849,
19.2484176034894,20.242765847194,21.2371140908985,22.231462334603,23.2258105783075,
24.220158822012,25.2145070657166,26.2088553094211,27.2032035531256,28.1975517968301,
29.1919000405346,30.1862482842392,31.1805965279437,32.1749447716482,33.1692930153527,
34.1636412590572,35.1579895027618,36.1523377464663,37.1466859901708,38.1410342338753,
39.1353824775798,40.1297307212843,41.1240789649889,42.1184272086934,43.1127754523979,
44.1071236961024,45.1014719398069,46.0958201835115,47.090168427216,48.0845166709205,
49.078864914625,50.0732131583295,51.0675614020341,52.0619096457386,53.0562578894431,
54.0506061331476,55.0449543768521,56.0393026205567,57.0336508642612,58.0279991079657,
59.0223473516702,60.0166955953747,61.0110438390793,62.0053920827838,62.9997403264883,
63.9940885701928,64.9884368138973,65.9827850576018,66.9771333013064,67.9714815450109,
68.9658297887154,69.9601780324199,70.9545262761244,71.948874519829,72.9432227635335,
73.937571007238,74.9319192509425,75.926267494647,76.9206157383516,77.9149639820561,
78.9093122257606,79.9036604694651),.UNSPECIFIED.);
#509=B_SPLINE_SURFACE_WITH_KNOTS('',3,3,((#37549,#37550,#37551,#37552,#37553,
#37554,#37555,#37556,#37557,#37558,#37559,#37560,#37561,#37562,#37563,#37564,
#37565,#37566,#37567,#37568,#37569,#37570,#37571,#37572,#37573,#37574,#37575,
#37576,#37577,#37578,#37579,#37580,#37581,#37582,#37583,#37584,#37585,#37586,
#37587,#37588,#37589,#37590,#37591,#37592,#37593,#37594,#37595,#37596,#37597,
#37598,#37599,#37600,#37601,#37602,#37603,#37604,#37605,#37606,#37607,#37608,
#37609,#37610,#37611,#37612,#37613,#37614,#37615,#37616,#37617,#37618,#37619,
#37620,#37621,#37622,#37623),(#37624,#37625,#37626,#37627,#37628,#37629,
#37630,#37631,#37632,#37633,#37634,#37635,#37636,#37637,#37638,#37639,#37640,
#37641,#37642,#37643,#37644,#37645,#37646,#37647,#37648,#37649,#37650,#37651,
#37652,#37653,#37654,#37655,#37656,#37657,#37658,#37659,#37660,#37661,#37662,
#37663,#37664,#37665,#37666,#37667,#37668,#37669,#37670,#37671,#37672,#37673,
#37674,#37675,#37676,#37677,#37678,#37679,#37680,#37681,#37682,#37683,#37684,
#37685,#37686,#37687,#37688,#37689,#37690,#37691,#37692,#37693,#37694,#37695,
#37696,#37697,#37698),(#37699,#37700,#37701,#37702,#37703,#37704,#37705,
#37706,#37707,#37708,#37709,#37710,#37711,#37712,#37713,#37714,#37715,#37716,
#37717,#37718,#37719,#37720,#37721,#37722,#37723,#37724,#37725,#37726,#37727,
#37728,#37729,#37730,#37731,#37732,#37733,#37734,#37735,#37736,#37737,#37738,
#37739,#37740,#37741,#37742,#37743,#37744,#37745,#37746,#37747,#37748,#37749,
#37750,#37751,#37752,#37753,#37754,#37755,#37756,#37757,#37758,#37759,#37760,
#37761,#37762,#37763,#37764,#37765,#37766,#37767,#37768,#37769,#37770,#37771,
#37772,#37773),(#37774,#37775,#37776,#37777,#37778,#37779,#37780,#37781,
#37782,#37783,#37784,#37785,#37786,#37787,#37788,#37789,#37790,#37791,#37792,
#37793,#37794,#37795,#37796,#37797,#37798,#37799,#37800,#37801,#37802,#37803,
#37804,#37805,#37806,#37807,#37808,#37809,#37810,#37811,#37812,#37813,#37814,
#37815,#37816,#37817,#37818,#37819,#37820,#37821,#37822,#37823,#37824,#37825,
#37826,#37827,#37828,#37829,#37830,#37831,#37832,#37833,#37834,#37835,#37836,
#37837,#37838,#37839,#37840,#37841,#37842,#37843,#37844,#37845,#37846,#37847,
#37848)),.UNSPECIFIED.,.F.,.F.,.F.,(4,4),(4,1,1,1,1,1,1,1,1,1,1,1,1,1,1,
1,1,1,1,1,1,1,1,1,1,1,1,1,1,1,1,1,1,1,1,1,1,1,1,1,1,1,1,1,1,1,1,1,1,1,1,
1,1,1,1,1,1,1,1,1,1,1,1,1,1,1,1,1,1,1,1,1,4),(0.,0.0460148164544132),(11.6154215191106,
12.6097697628151,13.6041180065196,14.5984662502242,15.5928144939287,16.5871627376332,
17.5815109813377,18.5758592250422,19.5702074687467,20.5645557124513,21.5589039561558,
22.5532521998603,23.5476004435648,24.5419486872693,25.5362969309739,26.5306451746784,
27.5249934183829,28.5193416620874,29.5136899057919,30.5080381494965,31.502386393201,
32.4967346369055,33.49108288061,34.4854311243145,35.4797793680191,36.4741276117236,
37.4684758554281,38.4628240991326,39.4571723428371,40.4515205865417,41.4458688302462,
42.4402170739507,43.4345653176552,44.4289135613597,45.4232618050643,46.4176100487688,
47.4119582924733,48.4063065361778,49.4006547798823,50.3950030235868,51.3893512672914,
52.3836995109959,53.3780477547004,54.3723959984049,55.3667442421094,56.361092485814,
57.3554407295185,58.349788973223,59.3441372169275,60.338485460632,61.3328337043366,
62.3271819480411,63.3215301917456,64.3158784354501,65.3102266791546,66.3045749228592,
67.2989231665637,68.2932714102682,69.2876196539727,70.2819678976772,71.2763161413818,
72.2706643850863,73.2650126287908,74.2593608724953,75.2537091161998,76.2480573599044,
77.2424056036089,78.2367538473134,79.2311020910179,80.2254503347224,81.2197985784269,
82.2141468221315,83.208495065836),.UNSPECIFIED.);
#825=B_SPLINE_CURVE_WITH_KNOTS('',3,(#36261,#36262,#36263,#36264,#36265,
#36266,#36267,#36268,#36269,#36270),.UNSPECIFIED.,.F.,.F.,(4,3,3,4),(-4.09254174883833,
-3.97739297481808,-2.98304473111356,-2.06514013327812),.UNSPECIFIED.);
#826=B_SPLINE_CURVE_WITH_KNOTS('',3,(#36273,#36274,#36275,#36276,#36277,
#36278,#36279),.UNSPECIFIED.,.F.,.F.,(4,3,4),(0.,0.994348243704517,1.11419103802957),
 .UNSPECIFIED.);
#827=B_SPLINE_CURVE_WITH_KNOTS('',3,(#36284,#36285,#36286,#36287,#36288,
#36289,#36290,#36291,#36292,#36293,#36294,#36295,#36296,#36297,#36298,#36299,
#36300,#36301,#36302,#36303,#36304,#36305),.UNSPECIFIED.,.F.,.F.,(4,3,3,
3,3,3,3,4),(-10.3757270560179,-9.9434824370452,-8.94913419334068,-7.95478594963616,
-6.96043770593164,-5.96608946222712,-4.9717412185226,-4.09254174883833),
 .UNSPECIFIED.);
#828=B_SPLINE_CURVE_WITH_KNOTS('',3,(#36306,#36307,#36308,#36309,#36310,
#36311,#36312,#36313,#36314,#36315,#36316,#36317,#36318,#36319,#36320,#36321,
#36322,#36323,#36324,#36325,#36326,#36327),.UNSPECIFIED.,.F.,.F.,(4,3,3,
3,3,3,3,4),(1.11419103802957,1.98869648740904,2.98304473111356,3.97739297481808,
4.9717412185226,5.96608946222712,6.96043770593164,7.39737634520915),
 .UNSPECIFIED.);
#829=B_SPLINE_CURVE_WITH_KNOTS('',3,(#36332,#36333,#36334,#36335,#36336,
#36337,#36338,#36339,#36340,#36341,#36342,#36343,#36344,#36345,#36346,#36347,
#36348,#36349,#36350,#36351,#36352,#36353),.UNSPECIFIED.,.F.,.F.,(4,3,3,
3,3,3,3,4),(-16.6589123631975,-15.9095718992723,-14.9152236555678,-13.9208754118633,
-12.9265271681588,-11.9321789244542,-10.9378306807497,-10.3757270560179),
 .UNSPECIFIED.);
#830=B_SPLINE_CURVE_WITH_KNOTS('',3,(#36354,#36355,#36356,#36357,#36358,
#36359,#36360,#36361,#36362,#36363,#36364,#36365,#36366,#36367,#36368,#36369,
#36370,#36371,#36372,#36373,#36374,#36375),.UNSPECIFIED.,.F.,.F.,(4,3,3,
3,3,3,3,4),(7.39737634520915,7.95478594963616,8.94913419334068,9.9434824370452,
10.9378306807497,11.9321789244542,12.9265271681588,13.6805616523887),
 .UNSPECIFIED.);
#831=B_SPLINE_CURVE_WITH_KNOTS('',3,(#36380,#36381,#36382,#36383,#36384,
#36385,#36386,#36387,#36388,#36389,#36390,#36391,#36392,#36393,#36394,#36395,
#36396,#36397,#36398,#36399,#36400,#36401,#36402,#36403,#36404),
 .UNSPECIFIED.,.F.,.F.,(4,3,3,3,3,3,3,3,4),(-22.9420976703771,-22.8700096052039,
-21.8756613614994,-20.8813131177949,-19.8869648740904,-18.8926166303859,
-17.8982683866814,-16.9039201429768,-16.6589123631975),.UNSPECIFIED.);
#832=B_SPLINE_CURVE_WITH_KNOTS('',3,(#36405,#36406,#36407,#36408,#36409,
#36410,#36411,#36412,#36413,#36414,#36415,#36416,#36417,#36418,#36419,#36420,
#36421,#36422,#36423,#36424,#36425,#36426,#36427,#36428,#36429),
 .UNSPECIFIED.,.F.,.F.,(4,3,3,3,3,3,3,3,4),(13.6805616523887,13.9208754118633,
14.9152236555678,15.9095718992723,16.9039201429768,17.8982683866814,18.8926166303859,
19.8869648740904,19.9637469595683),.UNSPECIFIED.);
#833=B_SPLINE_CURVE_WITH_KNOTS('',3,(#36434,#36435,#36436,#36437,#36438,
#36439,#36440,#36441,#36442,#36443,#36444,#36445,#36446,#36447,#36448,#36449,
#36450,#36451,#36452,#36453,#36454,#36455),.UNSPECIFIED.,.F.,.F.,(4,3,3,
3,3,3,3,4),(-29.2252829775567,-28.8360990674311,-27.8417508237265,-26.847402580022,
-25.8530543363175,-24.858706092613,-23.8643578489085,-22.9420976703771),
 .UNSPECIFIED.);
#834=B_SPLINE_CURVE_WITH_KNOTS('',3,(#36456,#36457,#36458,#36459,#36460,
#36461,#36462,#36463,#36464,#36465,#36466,#36467,#36468,#36469,#36470,#36471,
#36472,#36473,#36474,#36475,#36476,#36477),.UNSPECIFIED.,.F.,.F.,(4,3,3,
3,3,3,3,4),(19.9637469595683,20.8813131177949,21.8756613614994,22.8700096052039,
23.8643578489085,24.858706092613,25.8530543363175,26.2469322667479),
 .UNSPECIFIED.);
#835=B_SPLINE_CURVE_WITH_KNOTS('',3,(#36482,#36483,#36484,#36485,#36486,
#36487,#36488,#36489,#36490,#36491,#36492,#36493,#36494,#36495,#36496,#36497,
#36498,#36499,#36500,#36501,#36502,#36503),.UNSPECIFIED.,.F.,.F.,(4,3,3,
3,3,3,3,4),(-35.5084682847363,-34.8021885296582,-33.8078402859537,-32.8134920422491,
-31.8191437985446,-30.8247955548401,-29.8304473111356,-29.2252829775567),
 .UNSPECIFIED.);
#836=B_SPLINE_CURVE_WITH_KNOTS('',3,(#36504,#36505,#36506,#36507,#36508,
#36509,#36510,#36511,#36512,#36513,#36514,#36515,#36516,#36517,#36518,#36519,
#36520,#36521,#36522,#36523,#36524,#36525),.UNSPECIFIED.,.F.,.F.,(4,3,3,
3,3,3,3,4),(26.2469322667479,26.847402580022,27.8417508237265,28.8360990674311,
29.8304473111356,30.8247955548401,31.8191437985446,32.5301175739275),
 .UNSPECIFIED.);
#837=B_SPLINE_CURVE_WITH_KNOTS('',3,(#36530,#36531,#36532,#36533,#36534,
#36535,#36536,#36537,#36538,#36539,#36540,#36541,#36542,#36543,#36544,#36545,
#36546,#36547,#36548,#36549,#36550,#36551,#36552,#36553,#36554),
 .UNSPECIFIED.,.F.,.F.,(4,3,3,3,3,3,3,3,4),(-41.7916535919159,-41.7626262355898,
-40.7682779918853,-39.7739297481808,-38.7795815044762,-37.7852332607717,
-36.7908850170672,-35.7965367733627,-35.5084682847363),.UNSPECIFIED.);
#838=B_SPLINE_CURVE_WITH_KNOTS('',3,(#36555,#36556,#36557,#36558,#36559,
#36560,#36561,#36562,#36563,#36564,#36565,#36566,#36567,#36568,#36569,#36570,
#36571,#36572,#36573,#36574,#36575,#36576,#36577,#36578,#36579),
 .UNSPECIFIED.,.F.,.F.,(4,3,3,3,3,3,3,3,4),(32.5301175739275,32.8134920422491,
33.8078402859537,34.8021885296582,35.7965367733627,36.7908850170672,37.7852332607717,
38.7795815044763,38.8133028811071),.UNSPECIFIED.);
#839=B_SPLINE_CURVE_WITH_KNOTS('',3,(#36584,#36585,#36586,#36587,#36588,
#36589,#36590,#36591,#36592,#36593,#36594,#36595,#36596,#36597,#36598,#36599,
#36600,#36601,#36602,#36603,#36604,#36605),.UNSPECIFIED.,.F.,.F.,(4,3,3,
3,3,3,3,4),(-48.0748388990954,-47.7287156978169,-46.7343674541124,-45.7400192104079,
-44.7456709667034,-43.7513227229988,-42.7569744792943,-41.7916535919159),
 .UNSPECIFIED.);
#840=B_SPLINE_CURVE_WITH_KNOTS('',3,(#36606,#36607,#36608,#36609,#36610,
#36611,#36612,#36613,#36614,#36615,#36616,#36617,#36618,#36619,#36620,#36621,
#36622,#36623,#36624,#36625,#36626,#36627),.UNSPECIFIED.,.F.,.F.,(4,3,3,
3,3,3,3,4),(38.8133028811071,39.7739297481808,40.7682779918853,41.7626262355898,
42.7569744792943,43.7513227229989,44.7456709667034,45.0964881882867),
 .UNSPECIFIED.);
#841=B_SPLINE_CURVE_WITH_KNOTS('',3,(#36632,#36633,#36634,#36635,#36636,
#36637,#36638,#36639,#36640,#36641,#36642,#36643,#36644,#36645,#36646,#36647,
#36648,#36649,#36650,#36651,#36652,#36653),.UNSPECIFIED.,.F.,.F.,(4,3,3,
3,3,3,3,4),(-54.3580242062751,-53.694805160044,-52.7004569163395,-51.706108672635,
-50.7117604289305,-49.717412185226,-48.7230639415214,-48.0748388990954),
 .UNSPECIFIED.);
#842=B_SPLINE_CURVE_WITH_KNOTS('',3,(#36654,#36655,#36656,#36657,#36658,
#36659,#36660,#36661,#36662,#36663,#36664,#36665,#36666,#36667,#36668,#36669,
#36670,#36671,#36672,#36673,#36674,#36675),.UNSPECIFIED.,.F.,.F.,(4,3,3,
3,3,3,3,4),(45.0964881882867,45.7400192104079,46.7343674541124,47.7287156978169,
48.7230639415215,49.717412185226,50.7117604289305,51.3796734954663),
 .UNSPECIFIED.);
#843=B_SPLINE_CURVE_WITH_KNOTS('',3,(#36680,#36681,#36682,#36683,#36684,
#36685,#36686,#36687,#36688,#36689,#36690,#36691,#36692,#36693,#36694,#36695,
#36696,#36697,#36698,#36699,#36700,#36701),.UNSPECIFIED.,.F.,.F.,(4,3,3,
3,3,3,3,4),(-60.6412095134546,-59.6608946222712,-58.6665463785667,-57.6721981348621,
-56.6778498911576,-55.6835016474531,-54.6891534037486,-54.3580242062751),
 .UNSPECIFIED.);
#844=B_SPLINE_CURVE_WITH_KNOTS('',3,(#36702,#36703,#36704,#36705,#36706,
#36707,#36708,#36709,#36710,#36711,#36712,#36713,#36714,#36715,#36716,#36717,
#36718,#36719,#36720,#36721,#36722,#36723),.UNSPECIFIED.,.F.,.F.,(4,3,3,
3,3,3,3,4),(51.3796734954663,51.706108672635,52.7004569163395,53.6948051600441,
54.6891534037486,55.6835016474531,56.6778498911576,57.6628588026459),
 .UNSPECIFIED.);
#845=B_SPLINE_CURVE_WITH_KNOTS('',3,(#36728,#36729,#36730,#36731,#36732,
#36733,#36734,#36735,#36736,#36737,#36738,#36739,#36740,#36741,#36742,#36743,
#36744,#36745,#36746,#36747,#36748,#36749,#36750,#36751,#36752),
 .UNSPECIFIED.,.F.,.F.,(4,3,3,3,3,3,3,3,4),(-66.9243948206342,-66.6213323282028,
-65.6269840844983,-64.6326358407938,-63.6382875970892,-62.6439393533847,
-61.6495911096802,-60.6552428659757,-60.6412095134546),.UNSPECIFIED.);
#846=B_SPLINE_CURVE_WITH_KNOTS('',3,(#36753,#36754,#36755,#36756,#36757,
#36758,#36759,#36760,#36761,#36762,#36763,#36764,#36765,#36766,#36767,#36768,
#36769,#36770,#36771,#36772,#36773,#36774,#36775,#36776,#36777),
 .UNSPECIFIED.,.F.,.F.,(4,3,3,3,3,3,3,3,4),(57.6628588026459,57.6721981348621,
58.6665463785666,59.6608946222712,60.6552428659757,61.6495911096802,62.6439393533847,
63.6382875970892,63.9460441098255),.UNSPECIFIED.);
#847=B_SPLINE_CURVE_WITH_KNOTS('',3,(#36783,#36784,#36785,#36786,#36787,
#36788),.UNSPECIFIED.,.F.,.F.,(4,1,1,4),(78.5398163397449,79.2311020910179,
80.2254503347224,81.1433549325579),.UNSPECIFIED.);
#848=B_SPLINE_CURVE_WITH_KNOTS('',3,(#36791,#36792,#36793,#36794,#36795),
 .UNSPECIFIED.,.F.,.F.,(4,1,4),(78.5398163397448,78.9093122257606,79.9036604694651),
 .UNSPECIFIED.);
#849=B_SPLINE_CURVE_WITH_KNOTS('',3,(#36800,#36801,#36802,#36803,#36804,
#36805,#36806,#36807,#36808,#36809,#36810),.UNSPECIFIED.,.F.,.F.,(4,1,1,
1,1,1,1,1,4),(72.2566310325653,72.2706643850863,73.2650126287908,74.2593608724953,
75.2537091161998,76.2480573599044,77.2424056036089,78.2367538473134,78.5398163397449),
 .UNSPECIFIED.);
#850=B_SPLINE_CURVE_WITH_KNOTS('',3,(#36811,#36812,#36813,#36814,#36815,
#36816,#36817,#36818,#36819,#36820),.UNSPECIFIED.,.F.,.F.,(4,1,1,1,1,1,
1,4),(72.2566310325652,72.9432227635335,73.937571007238,74.9319192509425,
75.926267494647,76.9206157383516,77.9149639820561,78.5398163397448),
 .UNSPECIFIED.);
#851=B_SPLINE_CURVE_WITH_KNOTS('',3,(#36825,#36826,#36827,#36828,#36829,
#36830,#36831,#36832,#36833,#36834),.UNSPECIFIED.,.F.,.F.,(4,1,1,1,1,1,
1,4),(65.9734457253856,66.3045749228592,67.2989231665637,68.2932714102682,
69.2876196539727,70.2819678976772,71.2763161413818,72.2566310325653),
 .UNSPECIFIED.);
#852=B_SPLINE_CURVE_WITH_KNOTS('',3,(#36835,#36836,#36837,#36838,#36839,
#36840,#36841,#36842,#36843,#36844,#36845),.UNSPECIFIED.,.F.,.F.,(4,1,1,
1,1,1,1,1,4),(65.9734457253856,65.9827850576018,66.9771333013064,67.9714815450109,
68.9658297887154,69.9601780324199,70.9545262761244,71.948874519829,72.2566310325652),
 .UNSPECIFIED.);
#853=B_SPLINE_CURVE_WITH_KNOTS('',3,(#36850,#36851,#36852,#36853,#36854,
#36855,#36856,#36857,#36858,#36859),.UNSPECIFIED.,.F.,.F.,(4,1,1,1,1,1,
1,4),(59.6902604182061,60.338485460632,61.3328337043366,62.3271819480411,
63.3215301917456,64.3158784354501,65.3102266791546,65.9734457253856),
 .UNSPECIFIED.);
#854=B_SPLINE_CURVE_WITH_KNOTS('',3,(#36860,#36861,#36862,#36863,#36864,
#36865,#36866,#36867,#36868,#36869),.UNSPECIFIED.,.F.,.F.,(4,1,1,1,1,1,
1,4),(59.6902604182061,60.0166955953747,61.0110438390793,62.0053920827838,
62.9997403264883,63.9940885701928,64.9884368138973,65.9734457253856),
 .UNSPECIFIED.);
#855=B_SPLINE_CURVE_WITH_KNOTS('',3,(#36874,#36875,#36876,#36877,#36878,
#36879,#36880,#36881,#36882,#36883),.UNSPECIFIED.,.F.,.F.,(4,1,1,1,1,1,
1,4),(53.4070751110265,54.3723959984049,55.3667442421094,56.361092485814,
57.3554407295185,58.349788973223,59.3441372169275,59.6902604182061),
 .UNSPECIFIED.);
#856=B_SPLINE_CURVE_WITH_KNOTS('',3,(#36884,#36885,#36886,#36887,#36888,
#36889,#36890,#36891,#36892,#36893),.UNSPECIFIED.,.F.,.F.,(4,1,1,1,1,1,
1,4),(53.4070751110265,54.0506061331476,55.0449543768521,56.0393026205567,
57.0336508642612,58.0279991079657,59.0223473516702,59.6902604182061),
 .UNSPECIFIED.);
#857=B_SPLINE_CURVE_WITH_KNOTS('',3,(#36898,#36899,#36900,#36901,#36902,
#36903,#36904,#36905,#36906,#36907,#36908),.UNSPECIFIED.,.F.,.F.,(4,1,1,
1,1,1,1,1,4),(47.1238898038469,47.4119582924733,48.4063065361778,49.4006547798823,
50.3950030235868,51.3893512672914,52.3836995109959,53.3780477547004,53.4070751110265),
 .UNSPECIFIED.);
#858=B_SPLINE_CURVE_WITH_KNOTS('',3,(#36909,#36910,#36911,#36912,#36913,
#36914,#36915,#36916,#36917,#36918),.UNSPECIFIED.,.F.,.F.,(4,1,1,1,1,1,
1,4),(47.1238898038469,48.0845166709205,49.078864914625,50.0732131583295,
51.0675614020341,52.0619096457386,53.0562578894431,53.4070751110265),
 .UNSPECIFIED.);
#859=B_SPLINE_CURVE_WITH_KNOTS('',3,(#36923,#36924,#36925,#36926,#36927,
#36928,#36929,#36930,#36931,#36932),.UNSPECIFIED.,.F.,.F.,(4,1,1,1,1,1,
1,4),(40.8407044966673,41.4458688302462,42.4402170739507,43.4345653176552,
44.4289135613597,45.4232618050643,46.4176100487688,47.1238898038469),
 .UNSPECIFIED.);
#860=B_SPLINE_CURVE_WITH_KNOTS('',3,(#36933,#36934,#36935,#36936,#36937,
#36938,#36939,#36940,#36941,#36942,#36943),.UNSPECIFIED.,.F.,.F.,(4,1,1,
1,1,1,1,1,4),(40.8407044966673,41.1240789649889,42.1184272086934,43.1127754523979,
44.1071236961024,45.1014719398069,46.0958201835115,47.090168427216,47.1238898038469),
 .UNSPECIFIED.);
#861=B_SPLINE_CURVE_WITH_KNOTS('',3,(#36948,#36949,#36950,#36951,#36952,
#36953,#36954,#36955,#36956,#36957),.UNSPECIFIED.,.F.,.F.,(4,1,1,1,1,1,
1,4),(34.5575191894877,35.4797793680191,36.4741276117236,37.4684758554281,
38.4628240991326,39.4571723428371,40.4515205865417,40.8407044966673),
 .UNSPECIFIED.);
#862=B_SPLINE_CURVE_WITH_KNOTS('',3,(#36958,#36959,#36960,#36961,#36962,
#36963,#36964,#36965,#36966,#36967),.UNSPECIFIED.,.F.,.F.,(4,1,1,1,1,1,
1,4),(34.5575191894877,35.1579895027618,36.1523377464663,37.1466859901708,
38.1410342338753,39.1353824775798,40.1297307212843,40.8407044966673),
 .UNSPECIFIED.);
#863=B_SPLINE_CURVE_WITH_KNOTS('',3,(#36972,#36973,#36974,#36975,#36976,
#36977,#36978,#36979,#36980,#36981,#36982),.UNSPECIFIED.,.F.,.F.,(4,1,1,
1,1,1,1,1,4),(28.2743338823081,28.5193416620874,29.5136899057919,30.5080381494965,
31.502386393201,32.4967346369055,33.49108288061,34.4854311243145,34.5575191894877),
 .UNSPECIFIED.);
#864=B_SPLINE_CURVE_WITH_KNOTS('',3,(#36983,#36984,#36985,#36986,#36987,
#36988,#36989,#36990,#36991,#36992),.UNSPECIFIED.,.F.,.F.,(4,1,1,1,1,1,
1,4),(28.2743338823081,29.1919000405346,30.1862482842392,31.1805965279437,
32.1749447716482,33.1692930153527,34.1636412590572,34.5575191894877),
 .UNSPECIFIED.);
#865=B_SPLINE_CURVE_WITH_KNOTS('',3,(#36997,#36998,#36999,#37000,#37001,
#37002,#37003,#37004,#37005,#37006),.UNSPECIFIED.,.F.,.F.,(4,1,1,1,1,1,
1,4),(21.9911485751285,22.5532521998603,23.5476004435648,24.5419486872693,
25.5362969309739,26.5306451746784,27.5249934183829,28.2743338823081),
 .UNSPECIFIED.);
#866=B_SPLINE_CURVE_WITH_KNOTS('',3,(#37007,#37008,#37009,#37010,#37011,
#37012,#37013,#37014,#37015,#37016,#37017),.UNSPECIFIED.,.F.,.F.,(4,1,1,
1,1,1,1,1,4),(21.9911485751285,22.231462334603,23.2258105783075,24.220158822012,
25.2145070657166,26.2088553094211,27.2032035531256,28.1975517968301,28.2743338823081),
 .UNSPECIFIED.);
#867=B_SPLINE_CURVE_WITH_KNOTS('',3,(#37022,#37023,#37024,#37025,#37026,
#37027,#37028,#37029,#37030,#37031),.UNSPECIFIED.,.F.,.F.,(4,1,1,1,1,1,
1,4),(15.7079632679489,16.5871627376332,17.5815109813377,18.5758592250422,
19.5702074687467,20.5645557124513,21.5589039561558,21.9911485751285),
 .UNSPECIFIED.);
#868=B_SPLINE_CURVE_WITH_KNOTS('',3,(#37032,#37033,#37034,#37035,#37036,
#37037,#37038,#37039,#37040,#37041),.UNSPECIFIED.,.F.,.F.,(4,1,1,1,1,1,
1,4),(15.7079632679489,16.2653728723759,17.2597211160804,18.2540693597849,
19.2484176034894,20.242765847194,21.2371140908985,21.9911485751285),
 .UNSPECIFIED.);
#869=B_SPLINE_CURVE_WITH_KNOTS('',3,(#37343,#37344,#37345,#37346,#37347,
#37348,#37349,#37350,#37351,#37352,#37353,#37354,#37355,#37356,#37357,#37358,
#37359,#37360,#37361,#37362,#37363,#37364,#37365,#37366,#37367,#37368,#37369,
#37370,#37371,#37372,#37373,#37374,#37375,#37376,#37377,#37378,#37379,#37380,
#37381,#37382,#37383,#37384,#37385,#37386,#37387,#37388,#37389,#37390,#37391,
#37392,#37393,#37394,#37395,#37396,#37397),.UNSPECIFIED.,.F.,.F.,(4,3,3,
3,3,3,3,3,3,3,3,3,3,3,3,3,3,3,4),(-0.364629307890675,-0.34972378827242,
-0.322720263625586,-0.304347638378591,-0.283123644987568,-0.264601682105285,
-0.252328648782195,-0.215920039519477,-0.197925115950283,-0.186636791761712,
-0.165647166431853,-0.140760913934002,-0.127055807624798,-0.116187295826016,
-0.0871404718695121,-0.0682560541634265,-0.0546745507926151,-0.0223452933345784,
0.),.UNSPECIFIED.);
#870=B_SPLINE_CURVE_WITH_KNOTS('',3,(#37398,#37399,#37400,#37401,#37402,
#37403,#37404,#37405,#37406,#37407,#37408,#37409,#37410,#37411,#37412,#37413,
#37414,#37415,#37416),.UNSPECIFIED.,.F.,.F.,(4,3,3,3,3,3,4),(63.9460441098255,
64.6326358407938,65.6269840844983,66.6213323282028,67.6156805719073,68.6100288156118,
69.5279334134473),.UNSPECIFIED.);
#871=B_SPLINE_CURVE_WITH_KNOTS('',3,(#37418,#37419,#37420,#37421,#37422,
#37423,#37424,#37425,#37426,#37427,#37428,#37429,#37430,#37431,#37432,#37433,
#37434,#37435,#37436,#37437,#37438,#37439,#37440,#37441,#37442,#37443,#37444,
#37445,#37446,#37447,#37448,#37449,#37450,#37451,#37452,#37453,#37454,#37455,
#37456,#37457,#37458,#37459,#37460,#37461,#37462,#37463,#37464,#37465,#37466,
#37467,#37468,#37469),.UNSPECIFIED.,.F.,.F.,(4,3,3,3,3,3,3,3,3,3,3,3,3,
3,3,3,3,4),(-0.366397579005845,-0.354297286130077,-0.32692051483854,-0.315737482103616,
-0.289774380161196,-0.272943837084162,-0.237814929253474,-0.221139930607587,
-0.207673366759947,-0.18655652524636,-0.163236959590565,-0.1482203546737,
-0.138085786201687,-0.103564339651265,-0.0816322651568354,-0.0668657996484716,
-0.0283713742630058,0.),.UNSPECIFIED.);
#872=B_SPLINE_CURVE_WITH_KNOTS('',3,(#37470,#37471,#37472,#37473,#37474,
#37475,#37476,#37477,#37478),.UNSPECIFIED.,.F.,.F.,(4,1,1,1,1,1,4),(10.3757270560178,
11.2936316538533,12.2879798975578,13.2823281412623,14.2766763849668,15.2710246286714,
15.7079632679489),.UNSPECIFIED.);
#873=B_SPLINE_CURVE_WITH_KNOTS('',3,(#37484,#37485,#37486,#37487,#37488,
#37489,#37490,#37491,#37492,#37493,#37494,#37495,#37496,#37497,#37498,#37499,
#37500,#37501,#37502,#37503,#37504,#37505,#37506,#37507,#37508,#37509,#37510,
#37511,#37512,#37513,#37514,#37515,#37516,#37517,#37518,#37519,#37520,#37521,
#37522,#37523,#37524,#37525,#37526,#37527,#37528,#37529,#37530,#37531,#37532,
#37533,#37534,#37535,#37536,#37537,#37538),.UNSPECIFIED.,.F.,.F.,(4,3,3,
3,3,3,3,3,3,3,3,3,3,3,3,3,3,3,4),(-0.364629307890664,-0.349723788272418,
-0.32272025631553,-0.304347635918125,-0.283123621269396,-0.264601511160708,
-0.252328600826691,-0.2159199799845,-0.197925046601542,-0.186636790019817,
-0.165647166431849,-0.140761503006746,-0.127058155986358,-0.116187684714683,
-0.0871407635360122,-0.0682567232080817,-0.0546745590404074,-0.0223453321529391,
0.),.UNSPECIFIED.);
#874=B_SPLINE_CURVE_WITH_KNOTS('',3,(#37541,#37542,#37543,#37544,#37545,
#37546,#37547,#37548),.UNSPECIFIED.,.F.,.F.,(4,1,1,1,1,4),(11.6154215191106,
12.6097697628151,13.6041180065196,14.5984662502242,15.5928144939287,15.7079632679489),
 .UNSPECIFIED.);
#875=B_SPLINE_CURVE_WITH_KNOTS('',3,(#37850,#37851,#37852,#37853,#37854,
#37855,#37856,#37857,#37858,#37859,#37860,#37861,#37862,#37863,#37864,#37865,
#37866,#37867,#37868,#37869,#37870,#37871,#37872,#37873,#37874,#37875,#37876,
#37877,#37878,#37879,#37880,#37881,#37882,#37883,#37884,#37885,#37886,#37887,
#37888,#37889,#37890,#37891,#37892,#37893,#37894,#37895,#37896,#37897,#37898,
#37899,#37900,#37901),.UNSPECIFIED.,.F.,.F.,(4,3,3,3,3,3,3,3,3,3,3,3,3,
3,3,3,3,4),(-0.366397579005866,-0.354297286130098,-0.326920513926121,-0.315737475841804,
-0.28977472454701,-0.272943757381991,-0.237814845664656,-0.221139815084396,
-0.207673346380608,-0.186556525246364,-0.163236959590568,-0.148220372021337,
-0.138085817027126,-0.103564362770345,-0.0816323215052509,-0.0668658025503337,
-0.0283713861783979,0.),.UNSPECIFIED.);
#876=B_SPLINE_CURVE_WITH_KNOTS('',3,(#37902,#37903,#37904,#37905,#37906,
#37907,#37908,#37909,#37910,#37911,#37912,#37913,#37914,#37915,#37916,#37917),
 .UNSPECIFIED.,.F.,.F.,(4,3,3,3,3,4),(-71.5930735467254,-70.5987253030209,
-69.6043770593164,-68.6100288156118,-67.6156805719073,-66.9243948206342),
 .UNSPECIFIED.);
#1111=CYLINDRICAL_SURFACE('',#17624,0.1954);
#1112=CYLINDRICAL_SURFACE('',#17626,0.1954);
#1113=CYLINDRICAL_SURFACE('',#17627,0.1954);
#1114=CYLINDRICAL_SURFACE('',#17628,0.1954);
#1115=CYLINDRICAL_SURFACE('',#17629,0.1954);
#1116=CYLINDRICAL_SURFACE('',#17630,0.1954);
#1117=CYLINDRICAL_SURFACE('',#17631,0.1954);
#1118=CYLINDRICAL_SURFACE('',#17632,0.1954);
#1119=CYLINDRICAL_SURFACE('',#17633,0.1954);
#1120=CYLINDRICAL_SURFACE('',#17634,0.1954);
#1121=CYLINDRICAL_SURFACE('',#17635,0.1954);
#1122=CYLINDRICAL_SURFACE('',#17636,0.15555);
#1123=CYLINDRICAL_SURFACE('',#17638,0.15555);
#1124=CYLINDRICAL_SURFACE('',#17639,0.15555);
#1125=CYLINDRICAL_SURFACE('',#17640,0.15555);
#1126=CYLINDRICAL_SURFACE('',#17641,0.15555);
#1127=CYLINDRICAL_SURFACE('',#17642,0.15555);
#1128=CYLINDRICAL_SURFACE('',#17643,0.15555);
#1129=CYLINDRICAL_SURFACE('',#17644,0.15555);
#1130=CYLINDRICAL_SURFACE('',#17645,0.15555);
#1131=CYLINDRICAL_SURFACE('',#17646,0.15555);
#1132=CYLINDRICAL_SURFACE('',#17647,0.15555);
#1133=CYLINDRICAL_SURFACE('',#17652,0.15555);
#1134=CYLINDRICAL_SURFACE('',#17701,0.4);
#1135=CYLINDRICAL_SURFACE('',#17704,0.4);
#1136=CYLINDRICAL_SURFACE('',#17707,0.4);
#1137=CYLINDRICAL_SURFACE('',#17710,0.4);
#1138=CYLINDRICAL_SURFACE('',#17713,0.4);
#1139=CYLINDRICAL_SURFACE('',#17716,0.4);
#1140=CYLINDRICAL_SURFACE('',#17719,0.4);
#1141=CYLINDRICAL_SURFACE('',#17722,0.4);
#1142=CYLINDRICAL_SURFACE('',#17725,0.4);
#1143=CYLINDRICAL_SURFACE('',#17728,0.4);
#1144=CYLINDRICAL_SURFACE('',#17731,0.4);
#1145=CYLINDRICAL_SURFACE('',#17734,0.4);
#1146=CYLINDRICAL_SURFACE('',#17737,0.4);
#1147=CYLINDRICAL_SURFACE('',#17740,0.4);
#1148=CYLINDRICAL_SURFACE('',#17743,0.4);
#1149=CYLINDRICAL_SURFACE('',#17746,0.4);
#1150=CYLINDRICAL_SURFACE('',#17749,0.4);
#1151=CYLINDRICAL_SURFACE('',#17752,0.4);
#1152=CYLINDRICAL_SURFACE('',#17755,0.4);
#1153=CYLINDRICAL_SURFACE('',#17758,0.4);
#1154=CYLINDRICAL_SURFACE('',#17761,0.4);
#1155=CYLINDRICAL_SURFACE('',#17764,0.4);
#1156=CYLINDRICAL_SURFACE('',#17767,0.4);
#1157=CYLINDRICAL_SURFACE('',#17770,0.4);
#1158=CYLINDRICAL_SURFACE('',#17778,0.1954);
#1204=FACE_BOUND('',#3651,.T.);
#1615=CIRCLE('',#17625,0.1954);
#1616=CIRCLE('',#17637,0.15555);
#1617=CIRCLE('',#17649,0.1954);
#1618=CIRCLE('',#17650,0.1954);
#1619=CIRCLE('',#17651,0.15555);
#1620=CIRCLE('',#17702,0.4);
#1621=CIRCLE('',#17703,0.4);
#1622=CIRCLE('',#17705,0.4);
#1623=CIRCLE('',#17706,0.4);
#1624=CIRCLE('',#17708,0.4);
#1625=CIRCLE('',#17709,0.4);
#1626=CIRCLE('',#17711,0.4);
#1627=CIRCLE('',#17712,0.4);
#1628=CIRCLE('',#17714,0.4);
#1629=CIRCLE('',#17715,0.4);
#1630=CIRCLE('',#17717,0.4);
#1631=CIRCLE('',#17718,0.4);
#1632=CIRCLE('',#17720,0.4);
#1633=CIRCLE('',#17721,0.4);
#1634=CIRCLE('',#17723,0.4);
#1635=CIRCLE('',#17724,0.4);
#1636=CIRCLE('',#17726,0.4);
#1637=CIRCLE('',#17727,0.4);
#1638=CIRCLE('',#17729,0.4);
#1639=CIRCLE('',#17730,0.4);
#1640=CIRCLE('',#17732,0.4);
#1641=CIRCLE('',#17733,0.4);
#1642=CIRCLE('',#17735,0.4);
#1643=CIRCLE('',#17736,0.4);
#1644=CIRCLE('',#17738,0.4);
#1645=CIRCLE('',#17739,0.4);
#1646=CIRCLE('',#17741,0.4);
#1647=CIRCLE('',#17742,0.4);
#1648=CIRCLE('',#17744,0.4);
#1649=CIRCLE('',#17745,0.4);
#1650=CIRCLE('',#17747,0.4);
#1651=CIRCLE('',#17748,0.4);
#1652=CIRCLE('',#17750,0.4);
#1653=CIRCLE('',#17751,0.4);
#1654=CIRCLE('',#17753,0.4);
#1655=CIRCLE('',#17754,0.4);
#1656=CIRCLE('',#17756,0.4);
#1657=CIRCLE('',#17757,0.4);
#1658=CIRCLE('',#17759,0.4);
#1659=CIRCLE('',#17760,0.4);
#1660=CIRCLE('',#17762,0.4);
#1661=CIRCLE('',#17763,0.4);
#1662=CIRCLE('',#17765,0.4);
#1663=CIRCLE('',#17766,0.4);
#1664=CIRCLE('',#17768,0.4);
#1665=CIRCLE('',#17769,0.4);
#1666=CIRCLE('',#17771,0.4);
#1667=CIRCLE('',#17772,0.4);
#1668=CIRCLE('',#17774,0.36);
#1669=CIRCLE('',#17776,0.17);
#1670=CIRCLE('',#17779,0.1954);
#1671=CIRCLE('',#17782,0.35);
#1771=CONICAL_SURFACE('',#17773,0.38,0.785398163397449);
#1772=CONICAL_SURFACE('',#17777,0.185,0.785398163397448);
#1773=CONICAL_SURFACE('',#17781,0.375,0.785398163397449);
#2586=FACE_OUTER_BOUND('',#3548,.T.);
#2587=FACE_OUTER_BOUND('',#3549,.T.);
#2588=FACE_OUTER_BOUND('',#3550,.T.);
#2589=FACE_OUTER_BOUND('',#3551,.T.);
#2590=FACE_OUTER_BOUND('',#3552,.T.);
#2591=FACE_OUTER_BOUND('',#3553,.T.);
#2592=FACE_OUTER_BOUND('',#3554,.T.);
#2593=FACE_OUTER_BOUND('',#3555,.T.);
#2594=FACE_OUTER_BOUND('',#3556,.T.);
#2595=FACE_OUTER_BOUND('',#3557,.T.);
#2596=FACE_OUTER_BOUND('',#3558,.T.);
#2597=FACE_OUTER_BOUND('',#3559,.T.);
#2598=FACE_OUTER_BOUND('',#3560,.T.);
#2599=FACE_OUTER_BOUND('',#3561,.T.);
#2600=FACE_OUTER_BOUND('',#3562,.T.);
#2601=FACE_OUTER_BOUND('',#3563,.T.);
#2602=FACE_OUTER_BOUND('',#3564,.T.);
#2603=FACE_OUTER_BOUND('',#3565,.T.);
#2604=FACE_OUTER_BOUND('',#3566,.T.);
#2605=FACE_OUTER_BOUND('',#3567,.T.);
#2606=FACE_OUTER_BOUND('',#3568,.T.);
#2607=FACE_OUTER_BOUND('',#3569,.T.);
#2608=FACE_OUTER_BOUND('',#3570,.T.);
#2609=FACE_OUTER_BOUND('',#3571,.T.);
#2610=FACE_OUTER_BOUND('',#3572,.T.);
#2611=FACE_OUTER_BOUND('',#3573,.T.);
#2612=FACE_OUTER_BOUND('',#3574,.T.);
#2613=FACE_OUTER_BOUND('',#3575,.T.);
#2614=FACE_OUTER_BOUND('',#3576,.T.);
#2615=FACE_OUTER_BOUND('',#3577,.T.);
#2616=FACE_OUTER_BOUND('',#3578,.T.);
#2617=FACE_OUTER_BOUND('',#3579,.T.);
#2618=FACE_OUTER_BOUND('',#3580,.T.);
#2619=FACE_OUTER_BOUND('',#3581,.T.);
#2620=FACE_OUTER_BOUND('',#3582,.T.);
#2621=FACE_OUTER_BOUND('',#3583,.T.);
#2622=FACE_OUTER_BOUND('',#3584,.T.);
#2623=FACE_OUTER_BOUND('',#3585,.T.);
#2624=FACE_OUTER_BOUND('',#3586,.T.);
#2625=FACE_OUTER_BOUND('',#3587,.T.);
#2626=FACE_OUTER_BOUND('',#3588,.T.);
#2627=FACE_OUTER_BOUND('',#3589,.T.);
#2628=FACE_OUTER_BOUND('',#3590,.T.);
#2629=FACE_OUTER_BOUND('',#3591,.T.);
#2630=FACE_OUTER_BOUND('',#3592,.T.);
#2631=FACE_OUTER_BOUND('',#3593,.T.);
#2632=FACE_OUTER_BOUND('',#3594,.T.);
#2633=FACE_OUTER_BOUND('',#3595,.T.);
#2634=FACE_OUTER_BOUND('',#3596,.T.);
#2635=FACE_OUTER_BOUND('',#3597,.T.);
#2636=FACE_OUTER_BOUND('',#3598,.T.);
#2637=FACE_OUTER_BOUND('',#3599,.T.);
#2638=FACE_OUTER_BOUND('',#3600,.T.);
#2639=FACE_OUTER_BOUND('',#3601,.T.);
#2640=FACE_OUTER_BOUND('',#3602,.T.);
#2641=FACE_OUTER_BOUND('',#3603,.T.);
#2642=FACE_OUTER_BOUND('',#3604,.T.);
#2643=FACE_OUTER_BOUND('',#3605,.T.);
#2644=FACE_OUTER_BOUND('',#3606,.T.);
#2645=FACE_OUTER_BOUND('',#3607,.T.);
#2646=FACE_OUTER_BOUND('',#3608,.T.);
#2647=FACE_OUTER_BOUND('',#3609,.T.);
#2648=FACE_OUTER_BOUND('',#3610,.T.);
#2649=FACE_OUTER_BOUND('',#3611,.T.);
#2650=FACE_OUTER_BOUND('',#3612,.T.);
#2651=FACE_OUTER_BOUND('',#3613,.T.);
#2652=FACE_OUTER_BOUND('',#3614,.T.);
#2653=FACE_OUTER_BOUND('',#3615,.T.);
#2654=FACE_OUTER_BOUND('',#3616,.T.);
#2655=FACE_OUTER_BOUND('',#3617,.T.);
#2656=FACE_OUTER_BOUND('',#3618,.T.);
#2657=FACE_OUTER_BOUND('',#3619,.T.);
#2658=FACE_OUTER_BOUND('',#3620,.T.);
#2659=FACE_OUTER_BOUND('',#3621,.T.);
#2660=FACE_OUTER_BOUND('',#3622,.T.);
#2661=FACE_OUTER_BOUND('',#3623,.T.);
#2662=FACE_OUTER_BOUND('',#3624,.T.);
#2663=FACE_OUTER_BOUND('',#3625,.T.);
#2664=FACE_OUTER_BOUND('',#3626,.T.);
#2665=FACE_OUTER_BOUND('',#3627,.T.);
#2666=FACE_OUTER_BOUND('',#3628,.T.);
#2667=FACE_OUTER_BOUND('',#3629,.T.);
#2668=FACE_OUTER_BOUND('',#3630,.T.);
#2669=FACE_OUTER_BOUND('',#3631,.T.);
#2670=FACE_OUTER_BOUND('',#3632,.T.);
#2671=FACE_OUTER_BOUND('',#3633,.T.);
#2672=FACE_OUTER_BOUND('',#3634,.T.);
#2673=FACE_OUTER_BOUND('',#3635,.T.);
#2674=FACE_OUTER_BOUND('',#3636,.T.);
#2675=FACE_OUTER_BOUND('',#3637,.T.);
#2676=FACE_OUTER_BOUND('',#3638,.T.);
#2677=FACE_OUTER_BOUND('',#3639,.T.);
#2678=FACE_OUTER_BOUND('',#3640,.T.);
#2679=FACE_OUTER_BOUND('',#3641,.T.);
#2680=FACE_OUTER_BOUND('',#3642,.T.);
#2681=FACE_OUTER_BOUND('',#3643,.T.);
#2682=FACE_OUTER_BOUND('',#3644,.T.);
#2683=FACE_OUTER_BOUND('',#3645,.T.);
#2684=FACE_OUTER_BOUND('',#3646,.T.);
#2685=FACE_OUTER_BOUND('',#3647,.T.);
#2686=FACE_OUTER_BOUND('',#3648,.T.);
#2687=FACE_OUTER_BOUND('',#3649,.T.);
#2688=FACE_OUTER_BOUND('',#3650,.T.);
#2689=FACE_OUTER_BOUND('',#3652,.T.);
#2690=FACE_OUTER_BOUND('',#3653,.T.);
#3548=EDGE_LOOP('',(#14203,#14204,#14205,#14206));
#3549=EDGE_LOOP('',(#14207,#14208,#14209,#14210));
#3550=EDGE_LOOP('',(#14211,#14212,#14213,#14214));
#3551=EDGE_LOOP('',(#14215,#14216,#14217,#14218));
#3552=EDGE_LOOP('',(#14219,#14220,#14221,#14222));
#3553=EDGE_LOOP('',(#14223,#14224,#14225,#14226));
#3554=EDGE_LOOP('',(#14227,#14228,#14229,#14230));
#3555=EDGE_LOOP('',(#14231,#14232,#14233,#14234));
#3556=EDGE_LOOP('',(#14235,#14236,#14237,#14238));
#3557=EDGE_LOOP('',(#14239,#14240,#14241,#14242));
#3558=EDGE_LOOP('',(#14243,#14244,#14245,#14246));
#3559=EDGE_LOOP('',(#14247,#14248,#14249,#14250));
#3560=EDGE_LOOP('',(#14251,#14252,#14253,#14254));
#3561=EDGE_LOOP('',(#14255,#14256,#14257,#14258));
#3562=EDGE_LOOP('',(#14259,#14260,#14261,#14262));
#3563=EDGE_LOOP('',(#14263,#14264,#14265,#14266));
#3564=EDGE_LOOP('',(#14267,#14268,#14269,#14270));
#3565=EDGE_LOOP('',(#14271,#14272,#14273,#14274));
#3566=EDGE_LOOP('',(#14275,#14276,#14277,#14278));
#3567=EDGE_LOOP('',(#14279,#14280,#14281,#14282));
#3568=EDGE_LOOP('',(#14283,#14284,#14285,#14286));
#3569=EDGE_LOOP('',(#14287,#14288,#14289,#14290));
#3570=EDGE_LOOP('',(#14291,#14292,#14293,#14294,#14295,#14296,#14297,#14298,
#14299,#14300,#14301,#14302,#14303,#14304,#14305,#14306,#14307,#14308,#14309,
#14310,#14311,#14312,#14313,#14314,#14315,#14316));
#3571=EDGE_LOOP('',(#14317,#14318,#14319,#14320,#14321));
#3572=EDGE_LOOP('',(#14322,#14323,#14324,#14325));
#3573=EDGE_LOOP('',(#14326,#14327,#14328,#14329,#14330,#14331,#14332,#14333,
#14334,#14335,#14336,#14337,#14338,#14339,#14340,#14341,#14342,#14343,#14344,
#14345,#14346,#14347,#14348,#14349,#14350,#14351));
#3574=EDGE_LOOP('',(#14352,#14353,#14354,#14355));
#3575=EDGE_LOOP('',(#14356,#14357,#14358,#14359));
#3576=EDGE_LOOP('',(#14360,#14361,#14362,#14363));
#3577=EDGE_LOOP('',(#14364,#14365,#14366,#14367));
#3578=EDGE_LOOP('',(#14368,#14369,#14370,#14371));
#3579=EDGE_LOOP('',(#14372,#14373,#14374,#14375));
#3580=EDGE_LOOP('',(#14376,#14377,#14378,#14379));
#3581=EDGE_LOOP('',(#14380,#14381,#14382,#14383));
#3582=EDGE_LOOP('',(#14384,#14385,#14386,#14387));
#3583=EDGE_LOOP('',(#14388,#14389,#14390,#14391));
#3584=EDGE_LOOP('',(#14392,#14393,#14394,#14395));
#3585=EDGE_LOOP('',(#14396,#14397,#14398,#14399));
#3586=EDGE_LOOP('',(#14400,#14401,#14402,#14403));
#3587=EDGE_LOOP('',(#14404,#14405,#14406,#14407));
#3588=EDGE_LOOP('',(#14408,#14409,#14410,#14411));
#3589=EDGE_LOOP('',(#14412,#14413,#14414,#14415));
#3590=EDGE_LOOP('',(#14416,#14417,#14418,#14419));
#3591=EDGE_LOOP('',(#14420,#14421,#14422,#14423));
#3592=EDGE_LOOP('',(#14424,#14425,#14426,#14427));
#3593=EDGE_LOOP('',(#14428,#14429,#14430,#14431));
#3594=EDGE_LOOP('',(#14432,#14433,#14434,#14435));
#3595=EDGE_LOOP('',(#14436,#14437,#14438,#14439));
#3596=EDGE_LOOP('',(#14440,#14441,#14442,#14443));
#3597=EDGE_LOOP('',(#14444,#14445,#14446,#14447));
#3598=EDGE_LOOP('',(#14448,#14449,#14450,#14451));
#3599=EDGE_LOOP('',(#14452,#14453,#14454,#14455));
#3600=EDGE_LOOP('',(#14456,#14457,#14458,#14459));
#3601=EDGE_LOOP('',(#14460,#14461,#14462,#14463));
#3602=EDGE_LOOP('',(#14464,#14465,#14466,#14467));
#3603=EDGE_LOOP('',(#14468,#14469,#14470,#14471));
#3604=EDGE_LOOP('',(#14472,#14473,#14474,#14475));
#3605=EDGE_LOOP('',(#14476,#14477,#14478,#14479));
#3606=EDGE_LOOP('',(#14480,#14481,#14482,#14483));
#3607=EDGE_LOOP('',(#14484,#14485,#14486,#14487));
#3608=EDGE_LOOP('',(#14488,#14489,#14490,#14491));
#3609=EDGE_LOOP('',(#14492,#14493,#14494,#14495));
#3610=EDGE_LOOP('',(#14496,#14497,#14498,#14499));
#3611=EDGE_LOOP('',(#14500,#14501,#14502,#14503));
#3612=EDGE_LOOP('',(#14504,#14505,#14506,#14507));
#3613=EDGE_LOOP('',(#14508,#14509,#14510,#14511));
#3614=EDGE_LOOP('',(#14512,#14513,#14514,#14515));
#3615=EDGE_LOOP('',(#14516,#14517,#14518,#14519));
#3616=EDGE_LOOP('',(#14520,#14521,#14522,#14523));
#3617=EDGE_LOOP('',(#14524,#14525,#14526,#14527));
#3618=EDGE_LOOP('',(#14528,#14529,#14530,#14531));
#3619=EDGE_LOOP('',(#14532,#14533,#14534,#14535));
#3620=EDGE_LOOP('',(#14536,#14537,#14538,#14539));
#3621=EDGE_LOOP('',(#14540,#14541,#14542,#14543));
#3622=EDGE_LOOP('',(#14544,#14545,#14546,#14547));
#3623=EDGE_LOOP('',(#14548,#14549,#14550,#14551));
#3624=EDGE_LOOP('',(#14552,#14553,#14554,#14555));
#3625=EDGE_LOOP('',(#14556,#14557,#14558,#14559));
#3626=EDGE_LOOP('',(#14560,#14561,#14562,#14563));
#3627=EDGE_LOOP('',(#14564,#14565,#14566,#14567));
#3628=EDGE_LOOP('',(#14568,#14569,#14570,#14571));
#3629=EDGE_LOOP('',(#14572,#14573,#14574,#14575));
#3630=EDGE_LOOP('',(#14576,#14577,#14578,#14579));
#3631=EDGE_LOOP('',(#14580,#14581,#14582,#14583));
#3632=EDGE_LOOP('',(#14584,#14585,#14586,#14587));
#3633=EDGE_LOOP('',(#14588,#14589,#14590,#14591));
#3634=EDGE_LOOP('',(#14592,#14593,#14594,#14595));
#3635=EDGE_LOOP('',(#14596,#14597,#14598,#14599));
#3636=EDGE_LOOP('',(#14600,#14601,#14602,#14603));
#3637=EDGE_LOOP('',(#14604,#14605,#14606,#14607));
#3638=EDGE_LOOP('',(#14608,#14609,#14610,#14611));
#3639=EDGE_LOOP('',(#14612,#14613,#14614,#14615));
#3640=EDGE_LOOP('',(#14616,#14617,#14618,#14619));
#3641=EDGE_LOOP('',(#14620,#14621,#14622,#14623));
#3642=EDGE_LOOP('',(#14624,#14625,#14626,#14627));
#3643=EDGE_LOOP('',(#14628,#14629,#14630,#14631));
#3644=EDGE_LOOP('',(#14632,#14633,#14634,#14635));
#3645=EDGE_LOOP('',(#14636,#14637,#14638,#14639));
#3646=EDGE_LOOP('',(#14640,#14641,#14642,#14643,#14644,#14645,#14646,#14647,
#14648,#14649,#14650,#14651,#14652,#14653,#14654,#14655,#14656,#14657,#14658,
#14659,#14660,#14661,#14662,#14663,#14664,#14665,#14666,#14667,#14668,#14669,
#14670,#14671,#14672,#14673,#14674,#14675,#14676,#14677,#14678,#14679,#14680,
#14681,#14682,#14683,#14684,#14685,#14686,#14687,#14688,#14689,#14690,#14691,
#14692,#14693,#14694,#14695,#14696,#14697,#14698,#14699,#14700,#14701,#14702,
#14703,#14704,#14705,#14706,#14707,#14708,#14709,#14710,#14711,#14712,#14713,
#14714));
#3647=EDGE_LOOP('',(#14715));
#3648=EDGE_LOOP('',(#14716,#14717,#14718,#14719,#14720,#14721));
#3649=EDGE_LOOP('',(#14722,#14723,#14724,#14725));
#3650=EDGE_LOOP('',(#14726));
#3651=EDGE_LOOP('',(#14727,#14728,#14729,#14730));
#3652=EDGE_LOOP('',(#14731,#14732,#14733,#14734,#14735,#14736,#14737,#14738,
#14739,#14740,#14741,#14742,#14743,#14744,#14745,#14746,#14747,#14748,#14749,
#14750,#14751,#14752,#14753,#14754,#14755,#14756,#14757,#14758,#14759,#14760,
#14761,#14762,#14763,#14764,#14765,#14766,#14767,#14768,#14769,#14770,#14771,
#14772,#14773,#14774,#14775,#14776,#14777,#14778,#14779,#14780,#14781,#14782,
#14783,#14784,#14785,#14786,#14787,#14788,#14789,#14790,#14791,#14792,#14793,
#14794,#14795,#14796,#14797,#14798,#14799,#14800,#14801,#14802,#14803,#14804,
#14805));
#3653=EDGE_LOOP('',(#14806));
#4781=LINE('',#36259,#6005);
#4782=LINE('',#36283,#6006);
#4783=LINE('',#36331,#6007);
#4784=LINE('',#36379,#6008);
#4785=LINE('',#36433,#6009);
#4786=LINE('',#36481,#6010);
#4787=LINE('',#36529,#6011);
#4788=LINE('',#36583,#6012);
#4789=LINE('',#36631,#6013);
#4790=LINE('',#36679,#6014);
#4791=LINE('',#36727,#6015);
#4792=LINE('',#36781,#6016);
#4793=LINE('',#36799,#6017);
#4794=LINE('',#36824,#6018);
#4795=LINE('',#36849,#6019);
#4796=LINE('',#36873,#6020);
#4797=LINE('',#36897,#6021);
#4798=LINE('',#36922,#6022);
#4799=LINE('',#36947,#6023);
#4800=LINE('',#36971,#6024);
#4801=LINE('',#36996,#6025);
#4802=LINE('',#37021,#6026);
#4803=LINE('',#37925,#6027);
#4804=LINE('',#37930,#6028);
#4805=LINE('',#37937,#6029);
#4806=LINE('',#37948,#6030);
#4807=LINE('',#37953,#6031);
#4808=LINE('',#37960,#6032);
#4809=LINE('',#37971,#6033);
#4810=LINE('',#37976,#6034);
#4811=LINE('',#37983,#6035);
#4812=LINE('',#37994,#6036);
#4813=LINE('',#37999,#6037);
#4814=LINE('',#38006,#6038);
#4815=LINE('',#38017,#6039);
#4816=LINE('',#38022,#6040);
#4817=LINE('',#38029,#6041);
#4818=LINE('',#38040,#6042);
#4819=LINE('',#38045,#6043);
#4820=LINE('',#38052,#6044);
#4821=LINE('',#38063,#6045);
#4822=LINE('',#38068,#6046);
#4823=LINE('',#38075,#6047);
#4824=LINE('',#38086,#6048);
#4825=LINE('',#38091,#6049);
#4826=LINE('',#38098,#6050);
#4827=LINE('',#38109,#6051);
#4828=LINE('',#38114,#6052);
#4829=LINE('',#38121,#6053);
#4830=LINE('',#38132,#6054);
#4831=LINE('',#38137,#6055);
#4832=LINE('',#38144,#6056);
#4833=LINE('',#38155,#6057);
#4834=LINE('',#38160,#6058);
#4835=LINE('',#38167,#6059);
#4836=LINE('',#38178,#6060);
#4837=LINE('',#38183,#6061);
#4838=LINE('',#38190,#6062);
#4839=LINE('',#38201,#6063);
#4840=LINE('',#38206,#6064);
#4841=LINE('',#38213,#6065);
#4842=LINE('',#38224,#6066);
#4843=LINE('',#38229,#6067);
#4844=LINE('',#38236,#6068);
#4845=LINE('',#38247,#6069);
#4846=LINE('',#38252,#6070);
#4847=LINE('',#38259,#6071);
#4848=LINE('',#38270,#6072);
#4849=LINE('',#38275,#6073);
#4850=LINE('',#38282,#6074);
#4851=LINE('',#38293,#6075);
#4852=LINE('',#38298,#6076);
#4853=LINE('',#38305,#6077);
#4854=LINE('',#38316,#6078);
#4855=LINE('',#38321,#6079);
#4856=LINE('',#38328,#6080);
#4857=LINE('',#38339,#6081);
#4858=LINE('',#38344,#6082);
#4859=LINE('',#38351,#6083);
#4860=LINE('',#38362,#6084);
#4861=LINE('',#38367,#6085);
#4862=LINE('',#38374,#6086);
#4863=LINE('',#38385,#6087);
#4864=LINE('',#38390,#6088);
#4865=LINE('',#38397,#6089);
#4866=LINE('',#38408,#6090);
#4867=LINE('',#38413,#6091);
#4868=LINE('',#38420,#6092);
#4869=LINE('',#38431,#6093);
#4870=LINE('',#38436,#6094);
#4871=LINE('',#38443,#6095);
#4872=LINE('',#38454,#6096);
#4873=LINE('',#38459,#6097);
#4874=LINE('',#38466,#6098);
#4875=LINE('',#38544,#6099);
#4876=LINE('',#38550,#6100);
#4877=LINE('',#38557,#6101);
#6005=VECTOR('',#21376,0.2);
#6006=VECTOR('',#21381,0.2);
#6007=VECTOR('',#21384,0.2);
#6008=VECTOR('',#21387,0.2);
#6009=VECTOR('',#21390,0.2);
#6010=VECTOR('',#21393,0.2);
#6011=VECTOR('',#21396,0.2);
#6012=VECTOR('',#21399,0.2);
#6013=VECTOR('',#21402,0.2);
#6014=VECTOR('',#21405,0.2);
#6015=VECTOR('',#21408,0.2);
#6016=VECTOR('',#21411,0.15555);
#6017=VECTOR('',#21416,0.15555);
#6018=VECTOR('',#21419,0.15555);
#6019=VECTOR('',#21422,0.15555);
#6020=VECTOR('',#21425,0.15555);
#6021=VECTOR('',#21428,0.15555);
#6022=VECTOR('',#21431,0.15555);
#6023=VECTOR('',#21434,0.15555);
#6024=VECTOR('',#21437,0.15555);
#6025=VECTOR('',#21440,0.15555);
#6026=VECTOR('',#21443,0.15555);
#6027=VECTOR('',#21456,1.);
#6028=VECTOR('',#21457,1.);
#6029=VECTOR('',#21460,1.);
#6030=VECTOR('',#21463,1.);
#6031=VECTOR('',#21464,1.);
#6032=VECTOR('',#21467,1.);
#6033=VECTOR('',#21470,1.);
#6034=VECTOR('',#21471,1.);
#6035=VECTOR('',#21474,1.);
#6036=VECTOR('',#21477,1.);
#6037=VECTOR('',#21478,1.);
#6038=VECTOR('',#21481,1.);
#6039=VECTOR('',#21484,1.);
#6040=VECTOR('',#21485,1.);
#6041=VECTOR('',#21488,1.);
#6042=VECTOR('',#21491,1.);
#6043=VECTOR('',#21492,1.);
#6044=VECTOR('',#21495,1.);
#6045=VECTOR('',#21498,1.);
#6046=VECTOR('',#21499,1.);
#6047=VECTOR('',#21502,1.);
#6048=VECTOR('',#21505,1.);
#6049=VECTOR('',#21506,1.);
#6050=VECTOR('',#21509,1.);
#6051=VECTOR('',#21512,1.);
#6052=VECTOR('',#21513,1.);
#6053=VECTOR('',#21516,1.);
#6054=VECTOR('',#21519,1.);
#6055=VECTOR('',#21520,1.);
#6056=VECTOR('',#21523,1.);
#6057=VECTOR('',#21526,1.);
#6058=VECTOR('',#21527,1.);
#6059=VECTOR('',#21530,1.);
#6060=VECTOR('',#21533,1.);
#6061=VECTOR('',#21534,1.);
#6062=VECTOR('',#21537,1.);
#6063=VECTOR('',#21540,1.);
#6064=VECTOR('',#21541,1.);
#6065=VECTOR('',#21544,1.);
#6066=VECTOR('',#21547,1.);
#6067=VECTOR('',#21548,1.);
#6068=VECTOR('',#21551,1.);
#6069=VECTOR('',#21554,1.);
#6070=VECTOR('',#21555,1.);
#6071=VECTOR('',#21558,1.);
#6072=VECTOR('',#21561,1.);
#6073=VECTOR('',#21562,1.);
#6074=VECTOR('',#21565,1.);
#6075=VECTOR('',#21568,1.);
#6076=VECTOR('',#21569,1.);
#6077=VECTOR('',#21572,1.);
#6078=VECTOR('',#21575,1.);
#6079=VECTOR('',#21576,1.);
#6080=VECTOR('',#21579,1.);
#6081=VECTOR('',#21582,1.);
#6082=VECTOR('',#21583,1.);
#6083=VECTOR('',#21586,1.);
#6084=VECTOR('',#21589,1.);
#6085=VECTOR('',#21590,1.);
#6086=VECTOR('',#21593,1.);
#6087=VECTOR('',#21596,1.);
#6088=VECTOR('',#21597,1.);
#6089=VECTOR('',#21600,1.);
#6090=VECTOR('',#21603,1.);
#6091=VECTOR('',#21604,1.);
#6092=VECTOR('',#21607,1.);
#6093=VECTOR('',#21610,1.);
#6094=VECTOR('',#21611,1.);
#6095=VECTOR('',#21614,1.);
#6096=VECTOR('',#21617,1.);
#6097=VECTOR('',#21618,1.);
#6098=VECTOR('',#21621,1.);
#6099=VECTOR('',#21768,0.38);
#6100=VECTOR('',#21777,0.185);
#6101=VECTOR('',#21788,0.375);
#7425=VERTEX_POINT('',#36257);
#7426=VERTEX_POINT('',#36258);
#7427=VERTEX_POINT('',#36260);
#7428=VERTEX_POINT('',#36271);
#7429=VERTEX_POINT('',#36281);
#7430=VERTEX_POINT('',#36282);
#7431=VERTEX_POINT('',#36329);
#7432=VERTEX_POINT('',#36330);
#7433=VERTEX_POINT('',#36377);
#7434=VERTEX_POINT('',#36378);
#7435=VERTEX_POINT('',#36431);
#7436=VERTEX_POINT('',#36432);
#7437=VERTEX_POINT('',#36479);
#7438=VERTEX_POINT('',#36480);
#7439=VERTEX_POINT('',#36527);
#7440=VERTEX_POINT('',#36528);
#7441=VERTEX_POINT('',#36581);
#7442=VERTEX_POINT('',#36582);
#7443=VERTEX_POINT('',#36629);
#7444=VERTEX_POINT('',#36630);
#7445=VERTEX_POINT('',#36677);
#7446=VERTEX_POINT('',#36678);
#7447=VERTEX_POINT('',#36725);
#7448=VERTEX_POINT('',#36726);
#7449=VERTEX_POINT('',#36779);
#7450=VERTEX_POINT('',#36780);
#7451=VERTEX_POINT('',#36782);
#7452=VERTEX_POINT('',#36789);
#7453=VERTEX_POINT('',#36797);
#7454=VERTEX_POINT('',#36798);
#7455=VERTEX_POINT('',#36822);
#7456=VERTEX_POINT('',#36823);
#7457=VERTEX_POINT('',#36847);
#7458=VERTEX_POINT('',#36848);
#7459=VERTEX_POINT('',#36871);
#7460=VERTEX_POINT('',#36872);
#7461=VERTEX_POINT('',#36895);
#7462=VERTEX_POINT('',#36896);
#7463=VERTEX_POINT('',#36920);
#7464=VERTEX_POINT('',#36921);
#7465=VERTEX_POINT('',#36945);
#7466=VERTEX_POINT('',#36946);
#7467=VERTEX_POINT('',#36969);
#7468=VERTEX_POINT('',#36970);
#7469=VERTEX_POINT('',#36994);
#7470=VERTEX_POINT('',#36995);
#7471=VERTEX_POINT('',#37019);
#7472=VERTEX_POINT('',#37020);
#7473=VERTEX_POINT('',#37342);
#7474=VERTEX_POINT('',#37417);
#7475=VERTEX_POINT('',#37480);
#7476=VERTEX_POINT('',#37483);
#7477=VERTEX_POINT('',#37849);
#7478=VERTEX_POINT('',#37919);
#7479=VERTEX_POINT('',#37920);
#7480=VERTEX_POINT('',#37924);
#7481=VERTEX_POINT('',#37926);
#7482=VERTEX_POINT('',#37932);
#7483=VERTEX_POINT('',#37936);
#7484=VERTEX_POINT('',#37942);
#7485=VERTEX_POINT('',#37943);
#7486=VERTEX_POINT('',#37947);
#7487=VERTEX_POINT('',#37949);
#7488=VERTEX_POINT('',#37955);
#7489=VERTEX_POINT('',#37959);
#7490=VERTEX_POINT('',#37965);
#7491=VERTEX_POINT('',#37966);
#7492=VERTEX_POINT('',#37970);
#7493=VERTEX_POINT('',#37972);
#7494=VERTEX_POINT('',#37978);
#7495=VERTEX_POINT('',#37982);
#7496=VERTEX_POINT('',#37988);
#7497=VERTEX_POINT('',#37989);
#7498=VERTEX_POINT('',#37993);
#7499=VERTEX_POINT('',#37995);
#7500=VERTEX_POINT('',#38001);
#7501=VERTEX_POINT('',#38005);
#7502=VERTEX_POINT('',#38011);
#7503=VERTEX_POINT('',#38012);
#7504=VERTEX_POINT('',#38016);
#7505=VERTEX_POINT('',#38018);
#7506=VERTEX_POINT('',#38024);
#7507=VERTEX_POINT('',#38028);
#7508=VERTEX_POINT('',#38034);
#7509=VERTEX_POINT('',#38035);
#7510=VERTEX_POINT('',#38039);
#7511=VERTEX_POINT('',#38041);
#7512=VERTEX_POINT('',#38047);
#7513=VERTEX_POINT('',#38051);
#7514=VERTEX_POINT('',#38057);
#7515=VERTEX_POINT('',#38058);
#7516=VERTEX_POINT('',#38062);
#7517=VERTEX_POINT('',#38064);
#7518=VERTEX_POINT('',#38070);
#7519=VERTEX_POINT('',#38074);
#7520=VERTEX_POINT('',#38080);
#7521=VERTEX_POINT('',#38081);
#7522=VERTEX_POINT('',#38085);
#7523=VERTEX_POINT('',#38087);
#7524=VERTEX_POINT('',#38093);
#7525=VERTEX_POINT('',#38097);
#7526=VERTEX_POINT('',#38103);
#7527=VERTEX_POINT('',#38104);
#7528=VERTEX_POINT('',#38108);
#7529=VERTEX_POINT('',#38110);
#7530=VERTEX_POINT('',#38116);
#7531=VERTEX_POINT('',#38120);
#7532=VERTEX_POINT('',#38126);
#7533=VERTEX_POINT('',#38127);
#7534=VERTEX_POINT('',#38131);
#7535=VERTEX_POINT('',#38133);
#7536=VERTEX_POINT('',#38139);
#7537=VERTEX_POINT('',#38143);
#7538=VERTEX_POINT('',#38149);
#7539=VERTEX_POINT('',#38150);
#7540=VERTEX_POINT('',#38154);
#7541=VERTEX_POINT('',#38156);
#7542=VERTEX_POINT('',#38162);
#7543=VERTEX_POINT('',#38166);
#7544=VERTEX_POINT('',#38172);
#7545=VERTEX_POINT('',#38173);
#7546=VERTEX_POINT('',#38177);
#7547=VERTEX_POINT('',#38179);
#7548=VERTEX_POINT('',#38185);
#7549=VERTEX_POINT('',#38189);
#7550=VERTEX_POINT('',#38195);
#7551=VERTEX_POINT('',#38196);
#7552=VERTEX_POINT('',#38200);
#7553=VERTEX_POINT('',#38202);
#7554=VERTEX_POINT('',#38208);
#7555=VERTEX_POINT('',#38212);
#7556=VERTEX_POINT('',#38218);
#7557=VERTEX_POINT('',#38219);
#7558=VERTEX_POINT('',#38223);
#7559=VERTEX_POINT('',#38225);
#7560=VERTEX_POINT('',#38231);
#7561=VERTEX_POINT('',#38235);
#7562=VERTEX_POINT('',#38241);
#7563=VERTEX_POINT('',#38242);
#7564=VERTEX_POINT('',#38246);
#7565=VERTEX_POINT('',#38248);
#7566=VERTEX_POINT('',#38254);
#7567=VERTEX_POINT('',#38258);
#7568=VERTEX_POINT('',#38264);
#7569=VERTEX_POINT('',#38265);
#7570=VERTEX_POINT('',#38269);
#7571=VERTEX_POINT('',#38271);
#7572=VERTEX_POINT('',#38277);
#7573=VERTEX_POINT('',#38281);
#7574=VERTEX_POINT('',#38287);
#7575=VERTEX_POINT('',#38288);
#7576=VERTEX_POINT('',#38292);
#7577=VERTEX_POINT('',#38294);
#7578=VERTEX_POINT('',#38300);
#7579=VERTEX_POINT('',#38304);
#7580=VERTEX_POINT('',#38310);
#7581=VERTEX_POINT('',#38311);
#7582=VERTEX_POINT('',#38315);
#7583=VERTEX_POINT('',#38317);
#7584=VERTEX_POINT('',#38323);
#7585=VERTEX_POINT('',#38327);
#7586=VERTEX_POINT('',#38333);
#7587=VERTEX_POINT('',#38334);
#7588=VERTEX_POINT('',#38338);
#7589=VERTEX_POINT('',#38340);
#7590=VERTEX_POINT('',#38346);
#7591=VERTEX_POINT('',#38350);
#7592=VERTEX_POINT('',#38356);
#7593=VERTEX_POINT('',#38357);
#7594=VERTEX_POINT('',#38361);
#7595=VERTEX_POINT('',#38363);
#7596=VERTEX_POINT('',#38369);
#7597=VERTEX_POINT('',#38373);
#7598=VERTEX_POINT('',#38379);
#7599=VERTEX_POINT('',#38380);
#7600=VERTEX_POINT('',#38384);
#7601=VERTEX_POINT('',#38386);
#7602=VERTEX_POINT('',#38392);
#7603=VERTEX_POINT('',#38396);
#7604=VERTEX_POINT('',#38402);
#7605=VERTEX_POINT('',#38403);
#7606=VERTEX_POINT('',#38407);
#7607=VERTEX_POINT('',#38409);
#7608=VERTEX_POINT('',#38415);
#7609=VERTEX_POINT('',#38419);
#7610=VERTEX_POINT('',#38425);
#7611=VERTEX_POINT('',#38426);
#7612=VERTEX_POINT('',#38430);
#7613=VERTEX_POINT('',#38432);
#7614=VERTEX_POINT('',#38438);
#7615=VERTEX_POINT('',#38442);
#7616=VERTEX_POINT('',#38448);
#7617=VERTEX_POINT('',#38449);
#7618=VERTEX_POINT('',#38453);
#7619=VERTEX_POINT('',#38455);
#7620=VERTEX_POINT('',#38461);
#7621=VERTEX_POINT('',#38465);
#7622=VERTEX_POINT('',#38543);
#7623=VERTEX_POINT('',#38547);
#7624=VERTEX_POINT('',#38555);
#9717=EDGE_CURVE('',#7425,#7426,#4781,.T.);
#9718=EDGE_CURVE('',#7425,#7427,#825,.T.);
#9719=EDGE_CURVE('',#7427,#7428,#1615,.T.);
#9720=EDGE_CURVE('',#7428,#7426,#826,.T.);
#9721=EDGE_CURVE('',#7429,#7430,#4782,.T.);
#9722=EDGE_CURVE('',#7429,#7425,#827,.T.);
#9723=EDGE_CURVE('',#7426,#7430,#828,.T.);
#9724=EDGE_CURVE('',#7431,#7432,#4783,.T.);
#9725=EDGE_CURVE('',#7431,#7429,#829,.T.);
#9726=EDGE_CURVE('',#7430,#7432,#830,.T.);
#9727=EDGE_CURVE('',#7433,#7434,#4784,.T.);
#9728=EDGE_CURVE('',#7433,#7431,#831,.T.);
#9729=EDGE_CURVE('',#7432,#7434,#832,.T.);
#9730=EDGE_CURVE('',#7435,#7436,#4785,.T.);
#9731=EDGE_CURVE('',#7435,#7433,#833,.T.);
#9732=EDGE_CURVE('',#7434,#7436,#834,.T.);
#9733=EDGE_CURVE('',#7437,#7438,#4786,.T.);
#9734=EDGE_CURVE('',#7437,#7435,#835,.T.);
#9735=EDGE_CURVE('',#7436,#7438,#836,.T.);
#9736=EDGE_CURVE('',#7439,#7440,#4787,.T.);
#9737=EDGE_CURVE('',#7439,#7437,#837,.T.);
#9738=EDGE_CURVE('',#7438,#7440,#838,.T.);
#9739=EDGE_CURVE('',#7441,#7442,#4788,.T.);
#9740=EDGE_CURVE('',#7441,#7439,#839,.T.);
#9741=EDGE_CURVE('',#7440,#7442,#840,.T.);
#9742=EDGE_CURVE('',#7443,#7444,#4789,.T.);
#9743=EDGE_CURVE('',#7443,#7441,#841,.T.);
#9744=EDGE_CURVE('',#7442,#7444,#842,.T.);
#9745=EDGE_CURVE('',#7445,#7446,#4790,.T.);
#9746=EDGE_CURVE('',#7445,#7443,#843,.T.);
#9747=EDGE_CURVE('',#7444,#7446,#844,.T.);
#9748=EDGE_CURVE('',#7447,#7448,#4791,.T.);
#9749=EDGE_CURVE('',#7447,#7445,#845,.T.);
#9750=EDGE_CURVE('',#7446,#7448,#846,.T.);
#9751=EDGE_CURVE('',#7449,#7450,#4792,.T.);
#9752=EDGE_CURVE('',#7449,#7451,#847,.T.);
#9753=EDGE_CURVE('',#7452,#7451,#1616,.T.);
#9754=EDGE_CURVE('',#7450,#7452,#848,.T.);
#9755=EDGE_CURVE('',#7453,#7454,#4793,.T.);
#9756=EDGE_CURVE('',#7453,#7449,#849,.T.);
#9757=EDGE_CURVE('',#7454,#7450,#850,.T.);
#9758=EDGE_CURVE('',#7455,#7456,#4794,.T.);
#9759=EDGE_CURVE('',#7455,#7453,#851,.T.);
#9760=EDGE_CURVE('',#7456,#7454,#852,.T.);
#9761=EDGE_CURVE('',#7457,#7458,#4795,.T.);
#9762=EDGE_CURVE('',#7457,#7455,#853,.T.);
#9763=EDGE_CURVE('',#7458,#7456,#854,.T.);
#9764=EDGE_CURVE('',#7459,#7460,#4796,.T.);
#9765=EDGE_CURVE('',#7459,#7457,#855,.T.);
#9766=EDGE_CURVE('',#7460,#7458,#856,.T.);
#9767=EDGE_CURVE('',#7461,#7462,#4797,.T.);
#9768=EDGE_CURVE('',#7461,#7459,#857,.T.);
#9769=EDGE_CURVE('',#7462,#7460,#858,.T.);
#9770=EDGE_CURVE('',#7463,#7464,#4798,.T.);
#9771=EDGE_CURVE('',#7463,#7461,#859,.T.);
#9772=EDGE_CURVE('',#7464,#7462,#860,.T.);
#9773=EDGE_CURVE('',#7465,#7466,#4799,.T.);
#9774=EDGE_CURVE('',#7465,#7463,#861,.T.);
#9775=EDGE_CURVE('',#7466,#7464,#862,.T.);
#9776=EDGE_CURVE('',#7467,#7468,#4800,.T.);
#9777=EDGE_CURVE('',#7467,#7465,#863,.T.);
#9778=EDGE_CURVE('',#7468,#7466,#864,.T.);
#9779=EDGE_CURVE('',#7469,#7470,#4801,.T.);
#9780=EDGE_CURVE('',#7469,#7467,#865,.T.);
#9781=EDGE_CURVE('',#7470,#7468,#866,.T.);
#9782=EDGE_CURVE('',#7471,#7472,#4802,.T.);
#9783=EDGE_CURVE('',#7471,#7469,#867,.T.);
#9784=EDGE_CURVE('',#7472,#7470,#868,.T.);
#9785=EDGE_CURVE('',#7473,#7452,#869,.T.);
#9786=EDGE_CURVE('',#7448,#7473,#870,.T.);
#9787=EDGE_CURVE('',#7474,#7428,#871,.T.);
#9788=EDGE_CURVE('',#7474,#7472,#872,.T.);
#9789=EDGE_CURVE('',#7428,#7475,#1617,.T.);
#9790=EDGE_CURVE('',#7475,#7427,#1618,.T.);
#9791=EDGE_CURVE('',#7427,#7476,#873,.T.);
#9792=EDGE_CURVE('',#7476,#7474,#1619,.T.);
#9793=EDGE_CURVE('',#7476,#7471,#874,.T.);
#9794=EDGE_CURVE('',#7451,#7477,#875,.T.);
#9795=EDGE_CURVE('',#7477,#7447,#876,.T.);
#9796=EDGE_CURVE('',#7478,#7479,#336,.T.);
#9797=EDGE_CURVE('',#7478,#7480,#4803,.T.);
#9798=EDGE_CURVE('',#7481,#7480,#337,.T.);
#9799=EDGE_CURVE('',#7479,#7481,#4804,.T.);
#9800=EDGE_CURVE('',#7482,#7478,#338,.T.);
#9801=EDGE_CURVE('',#7483,#7482,#4805,.T.);
#9802=EDGE_CURVE('',#7480,#7483,#339,.T.);
#9803=EDGE_CURVE('',#7484,#7485,#340,.T.);
#9804=EDGE_CURVE('',#7484,#7486,#4806,.T.);
#9805=EDGE_CURVE('',#7487,#7486,#341,.T.);
#9806=EDGE_CURVE('',#7485,#7487,#4807,.T.);
#9807=EDGE_CURVE('',#7488,#7484,#342,.T.);
#9808=EDGE_CURVE('',#7489,#7488,#4808,.T.);
#9809=EDGE_CURVE('',#7486,#7489,#343,.T.);
#9810=EDGE_CURVE('',#7490,#7491,#344,.T.);
#9811=EDGE_CURVE('',#7490,#7492,#4809,.T.);
#9812=EDGE_CURVE('',#7493,#7492,#345,.T.);
#9813=EDGE_CURVE('',#7491,#7493,#4810,.T.);
#9814=EDGE_CURVE('',#7494,#7490,#346,.T.);
#9815=EDGE_CURVE('',#7495,#7494,#4811,.T.);
#9816=EDGE_CURVE('',#7492,#7495,#347,.T.);
#9817=EDGE_CURVE('',#7496,#7497,#348,.T.);
#9818=EDGE_CURVE('',#7496,#7498,#4812,.T.);
#9819=EDGE_CURVE('',#7499,#7498,#349,.T.);
#9820=EDGE_CURVE('',#7497,#7499,#4813,.T.);
#9821=EDGE_CURVE('',#7500,#7496,#350,.T.);
#9822=EDGE_CURVE('',#7501,#7500,#4814,.T.);
#9823=EDGE_CURVE('',#7498,#7501,#351,.T.);
#9824=EDGE_CURVE('',#7502,#7503,#352,.T.);
#9825=EDGE_CURVE('',#7502,#7504,#4815,.T.);
#9826=EDGE_CURVE('',#7505,#7504,#353,.T.);
#9827=EDGE_CURVE('',#7503,#7505,#4816,.T.);
#9828=EDGE_CURVE('',#7506,#7502,#354,.T.);
#9829=EDGE_CURVE('',#7507,#7506,#4817,.T.);
#9830=EDGE_CURVE('',#7504,#7507,#355,.T.);
#9831=EDGE_CURVE('',#7508,#7509,#356,.T.);
#9832=EDGE_CURVE('',#7508,#7510,#4818,.T.);
#9833=EDGE_CURVE('',#7511,#7510,#357,.T.);
#9834=EDGE_CURVE('',#7509,#7511,#4819,.T.);
#9835=EDGE_CURVE('',#7512,#7508,#358,.T.);
#9836=EDGE_CURVE('',#7513,#7512,#4820,.T.);
#9837=EDGE_CURVE('',#7510,#7513,#359,.T.);
#9838=EDGE_CURVE('',#7514,#7515,#360,.T.);
#9839=EDGE_CURVE('',#7514,#7516,#4821,.T.);
#9840=EDGE_CURVE('',#7517,#7516,#361,.T.);
#9841=EDGE_CURVE('',#7515,#7517,#4822,.T.);
#9842=EDGE_CURVE('',#7518,#7514,#362,.T.);
#9843=EDGE_CURVE('',#7519,#7518,#4823,.T.);
#9844=EDGE_CURVE('',#7516,#7519,#363,.T.);
#9845=EDGE_CURVE('',#7520,#7521,#364,.T.);
#9846=EDGE_CURVE('',#7520,#7522,#4824,.T.);
#9847=EDGE_CURVE('',#7523,#7522,#365,.T.);
#9848=EDGE_CURVE('',#7521,#7523,#4825,.T.);
#9849=EDGE_CURVE('',#7524,#7520,#366,.T.);
#9850=EDGE_CURVE('',#7525,#7524,#4826,.T.);
#9851=EDGE_CURVE('',#7522,#7525,#367,.T.);
#9852=EDGE_CURVE('',#7526,#7527,#368,.T.);
#9853=EDGE_CURVE('',#7526,#7528,#4827,.T.);
#9854=EDGE_CURVE('',#7529,#7528,#369,.T.);
#9855=EDGE_CURVE('',#7527,#7529,#4828,.T.);
#9856=EDGE_CURVE('',#7530,#7526,#370,.T.);
#9857=EDGE_CURVE('',#7531,#7530,#4829,.T.);
#9858=EDGE_CURVE('',#7528,#7531,#371,.T.);
#9859=EDGE_CURVE('',#7532,#7533,#372,.T.);
#9860=EDGE_CURVE('',#7532,#7534,#4830,.T.);
#9861=EDGE_CURVE('',#7535,#7534,#373,.T.);
#9862=EDGE_CURVE('',#7533,#7535,#4831,.T.);
#9863=EDGE_CURVE('',#7536,#7532,#374,.T.);
#9864=EDGE_CURVE('',#7537,#7536,#4832,.T.);
#9865=EDGE_CURVE('',#7534,#7537,#375,.T.);
#9866=EDGE_CURVE('',#7538,#7539,#376,.T.);
#9867=EDGE_CURVE('',#7538,#7540,#4833,.T.);
#9868=EDGE_CURVE('',#7541,#7540,#377,.T.);
#9869=EDGE_CURVE('',#7539,#7541,#4834,.T.);
#9870=EDGE_CURVE('',#7542,#7538,#378,.T.);
#9871=EDGE_CURVE('',#7543,#7542,#4835,.T.);
#9872=EDGE_CURVE('',#7540,#7543,#379,.T.);
#9873=EDGE_CURVE('',#7544,#7545,#380,.T.);
#9874=EDGE_CURVE('',#7544,#7546,#4836,.T.);
#9875=EDGE_CURVE('',#7547,#7546,#381,.T.);
#9876=EDGE_CURVE('',#7545,#7547,#4837,.T.);
#9877=EDGE_CURVE('',#7548,#7544,#382,.T.);
#9878=EDGE_CURVE('',#7549,#7548,#4838,.T.);
#9879=EDGE_CURVE('',#7546,#7549,#383,.T.);
#9880=EDGE_CURVE('',#7550,#7551,#384,.T.);
#9881=EDGE_CURVE('',#7550,#7552,#4839,.T.);
#9882=EDGE_CURVE('',#7553,#7552,#385,.T.);
#9883=EDGE_CURVE('',#7551,#7553,#4840,.T.);
#9884=EDGE_CURVE('',#7554,#7550,#386,.T.);
#9885=EDGE_CURVE('',#7555,#7554,#4841,.T.);
#9886=EDGE_CURVE('',#7552,#7555,#387,.T.);
#9887=EDGE_CURVE('',#7556,#7557,#388,.T.);
#9888=EDGE_CURVE('',#7556,#7558,#4842,.T.);
#9889=EDGE_CURVE('',#7559,#7558,#389,.T.);
#9890=EDGE_CURVE('',#7557,#7559,#4843,.T.);
#9891=EDGE_CURVE('',#7560,#7556,#390,.T.);
#9892=EDGE_CURVE('',#7561,#7560,#4844,.T.);
#9893=EDGE_CURVE('',#7558,#7561,#391,.T.);
#9894=EDGE_CURVE('',#7562,#7563,#392,.T.);
#9895=EDGE_CURVE('',#7562,#7564,#4845,.T.);
#9896=EDGE_CURVE('',#7565,#7564,#393,.T.);
#9897=EDGE_CURVE('',#7563,#7565,#4846,.T.);
#9898=EDGE_CURVE('',#7566,#7562,#394,.T.);
#9899=EDGE_CURVE('',#7567,#7566,#4847,.T.);
#9900=EDGE_CURVE('',#7564,#7567,#395,.T.);
#9901=EDGE_CURVE('',#7568,#7569,#396,.T.);
#9902=EDGE_CURVE('',#7568,#7570,#4848,.T.);
#9903=EDGE_CURVE('',#7571,#7570,#397,.T.);
#9904=EDGE_CURVE('',#7569,#7571,#4849,.T.);
#9905=EDGE_CURVE('',#7572,#7568,#398,.T.);
#9906=EDGE_CURVE('',#7573,#7572,#4850,.T.);
#9907=EDGE_CURVE('',#7570,#7573,#399,.T.);
#9908=EDGE_CURVE('',#7574,#7575,#400,.T.);
#9909=EDGE_CURVE('',#7574,#7576,#4851,.T.);
#9910=EDGE_CURVE('',#7577,#7576,#401,.T.);
#9911=EDGE_CURVE('',#7575,#7577,#4852,.T.);
#9912=EDGE_CURVE('',#7578,#7574,#402,.T.);
#9913=EDGE_CURVE('',#7579,#7578,#4853,.T.);
#9914=EDGE_CURVE('',#7576,#7579,#403,.T.);
#9915=EDGE_CURVE('',#7580,#7581,#404,.T.);
#9916=EDGE_CURVE('',#7580,#7582,#4854,.T.);
#9917=EDGE_CURVE('',#7583,#7582,#405,.T.);
#9918=EDGE_CURVE('',#7581,#7583,#4855,.T.);
#9919=EDGE_CURVE('',#7584,#7580,#406,.T.);
#9920=EDGE_CURVE('',#7585,#7584,#4856,.T.);
#9921=EDGE_CURVE('',#7582,#7585,#407,.T.);
#9922=EDGE_CURVE('',#7586,#7587,#408,.T.);
#9923=EDGE_CURVE('',#7586,#7588,#4857,.T.);
#9924=EDGE_CURVE('',#7589,#7588,#409,.T.);
#9925=EDGE_CURVE('',#7587,#7589,#4858,.T.);
#9926=EDGE_CURVE('',#7590,#7586,#410,.T.);
#9927=EDGE_CURVE('',#7591,#7590,#4859,.T.);
#9928=EDGE_CURVE('',#7588,#7591,#411,.T.);
#9929=EDGE_CURVE('',#7592,#7593,#412,.T.);
#9930=EDGE_CURVE('',#7592,#7594,#4860,.T.);
#9931=EDGE_CURVE('',#7595,#7594,#413,.T.);
#9932=EDGE_CURVE('',#7593,#7595,#4861,.T.);
#9933=EDGE_CURVE('',#7596,#7592,#414,.T.);
#9934=EDGE_CURVE('',#7597,#7596,#4862,.T.);
#9935=EDGE_CURVE('',#7594,#7597,#415,.T.);
#9936=EDGE_CURVE('',#7598,#7599,#416,.T.);
#9937=EDGE_CURVE('',#7598,#7600,#4863,.T.);
#9938=EDGE_CURVE('',#7601,#7600,#417,.T.);
#9939=EDGE_CURVE('',#7599,#7601,#4864,.T.);
#9940=EDGE_CURVE('',#7602,#7598,#418,.T.);
#9941=EDGE_CURVE('',#7603,#7602,#4865,.T.);
#9942=EDGE_CURVE('',#7600,#7603,#419,.T.);
#9943=EDGE_CURVE('',#7604,#7605,#420,.T.);
#9944=EDGE_CURVE('',#7604,#7606,#4866,.T.);
#9945=EDGE_CURVE('',#7607,#7606,#421,.T.);
#9946=EDGE_CURVE('',#7605,#7607,#4867,.T.);
#9947=EDGE_CURVE('',#7608,#7604,#422,.T.);
#9948=EDGE_CURVE('',#7609,#7608,#4868,.T.);
#9949=EDGE_CURVE('',#7606,#7609,#423,.T.);
#9950=EDGE_CURVE('',#7610,#7611,#424,.T.);
#9951=EDGE_CURVE('',#7610,#7612,#4869,.T.);
#9952=EDGE_CURVE('',#7613,#7612,#425,.T.);
#9953=EDGE_CURVE('',#7611,#7613,#4870,.T.);
#9954=EDGE_CURVE('',#7614,#7610,#426,.T.);
#9955=EDGE_CURVE('',#7615,#7614,#4871,.T.);
#9956=EDGE_CURVE('',#7612,#7615,#427,.T.);
#9957=EDGE_CURVE('',#7616,#7617,#428,.T.);
#9958=EDGE_CURVE('',#7616,#7618,#4872,.T.);
#9959=EDGE_CURVE('',#7619,#7618,#429,.T.);
#9960=EDGE_CURVE('',#7617,#7619,#4873,.T.);
#9961=EDGE_CURVE('',#7620,#7616,#430,.T.);
#9962=EDGE_CURVE('',#7621,#7620,#4874,.T.);
#9963=EDGE_CURVE('',#7618,#7621,#431,.T.);
#9964=EDGE_CURVE('',#7617,#7584,#1620,.T.);
#9965=EDGE_CURVE('',#7619,#7585,#1621,.T.);
#9966=EDGE_CURVE('',#7581,#7548,#1622,.T.);
#9967=EDGE_CURVE('',#7583,#7549,#1623,.T.);
#9968=EDGE_CURVE('',#7547,#7555,#1624,.T.);
#9969=EDGE_CURVE('',#7545,#7554,#1625,.T.);
#9970=EDGE_CURVE('',#7551,#7542,#1626,.T.);
#9971=EDGE_CURVE('',#7553,#7543,#1627,.T.);
#9972=EDGE_CURVE('',#7541,#7561,#1628,.T.);
#9973=EDGE_CURVE('',#7539,#7560,#1629,.T.);
#9974=EDGE_CURVE('',#7557,#7536,#1630,.T.);
#9975=EDGE_CURVE('',#7559,#7537,#1631,.T.);
#9976=EDGE_CURVE('',#7535,#7567,#1632,.T.);
#9977=EDGE_CURVE('',#7533,#7566,#1633,.T.);
#9978=EDGE_CURVE('',#7563,#7530,#1634,.T.);
#9979=EDGE_CURVE('',#7565,#7531,#1635,.T.);
#9980=EDGE_CURVE('',#7529,#7573,#1636,.T.);
#9981=EDGE_CURVE('',#7527,#7572,#1637,.T.);
#9982=EDGE_CURVE('',#7569,#7524,#1638,.T.);
#9983=EDGE_CURVE('',#7571,#7525,#1639,.T.);
#9984=EDGE_CURVE('',#7523,#7579,#1640,.T.);
#9985=EDGE_CURVE('',#7521,#7578,#1641,.T.);
#9986=EDGE_CURVE('',#7575,#7518,#1642,.T.);
#9987=EDGE_CURVE('',#7577,#7519,#1643,.T.);
#9988=EDGE_CURVE('',#7515,#7512,#1644,.T.);
#9989=EDGE_CURVE('',#7517,#7513,#1645,.T.);
#9990=EDGE_CURVE('',#7511,#7591,#1646,.T.);
#9991=EDGE_CURVE('',#7509,#7590,#1647,.T.);
#9992=EDGE_CURVE('',#7587,#7506,#1648,.T.);
#9993=EDGE_CURVE('',#7589,#7507,#1649,.T.);
#9994=EDGE_CURVE('',#7505,#7597,#1650,.T.);
#9995=EDGE_CURVE('',#7503,#7596,#1651,.T.);
#9996=EDGE_CURVE('',#7593,#7500,#1652,.T.);
#9997=EDGE_CURVE('',#7595,#7501,#1653,.T.);
#9998=EDGE_CURVE('',#7499,#7603,#1654,.T.);
#9999=EDGE_CURVE('',#7497,#7602,#1655,.T.);
#10000=EDGE_CURVE('',#7599,#7494,#1656,.T.);
#10001=EDGE_CURVE('',#7601,#7495,#1657,.T.);
#10002=EDGE_CURVE('',#7493,#7609,#1658,.T.);
#10003=EDGE_CURVE('',#7491,#7608,#1659,.T.);
#10004=EDGE_CURVE('',#7605,#7488,#1660,.T.);
#10005=EDGE_CURVE('',#7607,#7489,#1661,.T.);
#10006=EDGE_CURVE('',#7487,#7615,#1662,.T.);
#10007=EDGE_CURVE('',#7485,#7614,#1663,.T.);
#10008=EDGE_CURVE('',#7611,#7482,#1664,.T.);
#10009=EDGE_CURVE('',#7613,#7483,#1665,.T.);
#10010=EDGE_CURVE('',#7481,#7621,#1666,.T.);
#10011=EDGE_CURVE('',#7479,#7620,#1667,.T.);
#10012=EDGE_CURVE('',#7510,#7622,#4875,.T.);
#10013=EDGE_CURVE('',#7622,#7622,#1668,.T.);
#10014=EDGE_CURVE('',#7623,#7623,#1669,.T.);
#10015=EDGE_CURVE('',#7475,#7623,#4876,.T.);
#10016=EDGE_CURVE('',#7477,#7473,#1670,.T.);
#10017=EDGE_CURVE('',#7624,#7624,#1671,.T.);
#10018=EDGE_CURVE('',#7624,#7508,#4877,.T.);
#14203=ORIENTED_EDGE('',*,*,#9717,.F.);
#14204=ORIENTED_EDGE('',*,*,#9718,.T.);
#14205=ORIENTED_EDGE('',*,*,#9719,.T.);
#14206=ORIENTED_EDGE('',*,*,#9720,.T.);
#14207=ORIENTED_EDGE('',*,*,#9721,.F.);
#14208=ORIENTED_EDGE('',*,*,#9722,.T.);
#14209=ORIENTED_EDGE('',*,*,#9717,.T.);
#14210=ORIENTED_EDGE('',*,*,#9723,.T.);
#14211=ORIENTED_EDGE('',*,*,#9724,.F.);
#14212=ORIENTED_EDGE('',*,*,#9725,.T.);
#14213=ORIENTED_EDGE('',*,*,#9721,.T.);
#14214=ORIENTED_EDGE('',*,*,#9726,.T.);
#14215=ORIENTED_EDGE('',*,*,#9727,.F.);
#14216=ORIENTED_EDGE('',*,*,#9728,.T.);
#14217=ORIENTED_EDGE('',*,*,#9724,.T.);
#14218=ORIENTED_EDGE('',*,*,#9729,.T.);
#14219=ORIENTED_EDGE('',*,*,#9730,.F.);
#14220=ORIENTED_EDGE('',*,*,#9731,.T.);
#14221=ORIENTED_EDGE('',*,*,#9727,.T.);
#14222=ORIENTED_EDGE('',*,*,#9732,.T.);
#14223=ORIENTED_EDGE('',*,*,#9733,.F.);
#14224=ORIENTED_EDGE('',*,*,#9734,.T.);
#14225=ORIENTED_EDGE('',*,*,#9730,.T.);
#14226=ORIENTED_EDGE('',*,*,#9735,.T.);
#14227=ORIENTED_EDGE('',*,*,#9736,.F.);
#14228=ORIENTED_EDGE('',*,*,#9737,.T.);
#14229=ORIENTED_EDGE('',*,*,#9733,.T.);
#14230=ORIENTED_EDGE('',*,*,#9738,.T.);
#14231=ORIENTED_EDGE('',*,*,#9739,.F.);
#14232=ORIENTED_EDGE('',*,*,#9740,.T.);
#14233=ORIENTED_EDGE('',*,*,#9736,.T.);
#14234=ORIENTED_EDGE('',*,*,#9741,.T.);
#14235=ORIENTED_EDGE('',*,*,#9742,.F.);
#14236=ORIENTED_EDGE('',*,*,#9743,.T.);
#14237=ORIENTED_EDGE('',*,*,#9739,.T.);
#14238=ORIENTED_EDGE('',*,*,#9744,.T.);
#14239=ORIENTED_EDGE('',*,*,#9745,.F.);
#14240=ORIENTED_EDGE('',*,*,#9746,.T.);
#14241=ORIENTED_EDGE('',*,*,#9742,.T.);
#14242=ORIENTED_EDGE('',*,*,#9747,.T.);
#14243=ORIENTED_EDGE('',*,*,#9748,.F.);
#14244=ORIENTED_EDGE('',*,*,#9749,.T.);
#14245=ORIENTED_EDGE('',*,*,#9745,.T.);
#14246=ORIENTED_EDGE('',*,*,#9750,.T.);
#14247=ORIENTED_EDGE('',*,*,#9751,.F.);
#14248=ORIENTED_EDGE('',*,*,#9752,.T.);
#14249=ORIENTED_EDGE('',*,*,#9753,.F.);
#14250=ORIENTED_EDGE('',*,*,#9754,.F.);
#14251=ORIENTED_EDGE('',*,*,#9755,.F.);
#14252=ORIENTED_EDGE('',*,*,#9756,.T.);
#14253=ORIENTED_EDGE('',*,*,#9751,.T.);
#14254=ORIENTED_EDGE('',*,*,#9757,.F.);
#14255=ORIENTED_EDGE('',*,*,#9758,.F.);
#14256=ORIENTED_EDGE('',*,*,#9759,.T.);
#14257=ORIENTED_EDGE('',*,*,#9755,.T.);
#14258=ORIENTED_EDGE('',*,*,#9760,.F.);
#14259=ORIENTED_EDGE('',*,*,#9761,.F.);
#14260=ORIENTED_EDGE('',*,*,#9762,.T.);
#14261=ORIENTED_EDGE('',*,*,#9758,.T.);
#14262=ORIENTED_EDGE('',*,*,#9763,.F.);
#14263=ORIENTED_EDGE('',*,*,#9764,.F.);
#14264=ORIENTED_EDGE('',*,*,#9765,.T.);
#14265=ORIENTED_EDGE('',*,*,#9761,.T.);
#14266=ORIENTED_EDGE('',*,*,#9766,.F.);
#14267=ORIENTED_EDGE('',*,*,#9767,.F.);
#14268=ORIENTED_EDGE('',*,*,#9768,.T.);
#14269=ORIENTED_EDGE('',*,*,#9764,.T.);
#14270=ORIENTED_EDGE('',*,*,#9769,.F.);
#14271=ORIENTED_EDGE('',*,*,#9770,.F.);
#14272=ORIENTED_EDGE('',*,*,#9771,.T.);
#14273=ORIENTED_EDGE('',*,*,#9767,.T.);
#14274=ORIENTED_EDGE('',*,*,#9772,.F.);
#14275=ORIENTED_EDGE('',*,*,#9773,.F.);
#14276=ORIENTED_EDGE('',*,*,#9774,.T.);
#14277=ORIENTED_EDGE('',*,*,#9770,.T.);
#14278=ORIENTED_EDGE('',*,*,#9775,.F.);
#14279=ORIENTED_EDGE('',*,*,#9776,.F.);
#14280=ORIENTED_EDGE('',*,*,#9777,.T.);
#14281=ORIENTED_EDGE('',*,*,#9773,.T.);
#14282=ORIENTED_EDGE('',*,*,#9778,.F.);
#14283=ORIENTED_EDGE('',*,*,#9779,.F.);
#14284=ORIENTED_EDGE('',*,*,#9780,.T.);
#14285=ORIENTED_EDGE('',*,*,#9776,.T.);
#14286=ORIENTED_EDGE('',*,*,#9781,.F.);
#14287=ORIENTED_EDGE('',*,*,#9782,.F.);
#14288=ORIENTED_EDGE('',*,*,#9783,.T.);
#14289=ORIENTED_EDGE('',*,*,#9779,.T.);
#14290=ORIENTED_EDGE('',*,*,#9784,.F.);
#14291=ORIENTED_EDGE('',*,*,#9785,.F.);
#14292=ORIENTED_EDGE('',*,*,#9786,.F.);
#14293=ORIENTED_EDGE('',*,*,#9750,.F.);
#14294=ORIENTED_EDGE('',*,*,#9747,.F.);
#14295=ORIENTED_EDGE('',*,*,#9744,.F.);
#14296=ORIENTED_EDGE('',*,*,#9741,.F.);
#14297=ORIENTED_EDGE('',*,*,#9738,.F.);
#14298=ORIENTED_EDGE('',*,*,#9735,.F.);
#14299=ORIENTED_EDGE('',*,*,#9732,.F.);
#14300=ORIENTED_EDGE('',*,*,#9729,.F.);
#14301=ORIENTED_EDGE('',*,*,#9726,.F.);
#14302=ORIENTED_EDGE('',*,*,#9723,.F.);
#14303=ORIENTED_EDGE('',*,*,#9720,.F.);
#14304=ORIENTED_EDGE('',*,*,#9787,.F.);
#14305=ORIENTED_EDGE('',*,*,#9788,.T.);
#14306=ORIENTED_EDGE('',*,*,#9784,.T.);
#14307=ORIENTED_EDGE('',*,*,#9781,.T.);
#14308=ORIENTED_EDGE('',*,*,#9778,.T.);
#14309=ORIENTED_EDGE('',*,*,#9775,.T.);
#14310=ORIENTED_EDGE('',*,*,#9772,.T.);
#14311=ORIENTED_EDGE('',*,*,#9769,.T.);
#14312=ORIENTED_EDGE('',*,*,#9766,.T.);
#14313=ORIENTED_EDGE('',*,*,#9763,.T.);
#14314=ORIENTED_EDGE('',*,*,#9760,.T.);
#14315=ORIENTED_EDGE('',*,*,#9757,.T.);
#14316=ORIENTED_EDGE('',*,*,#9754,.T.);
#14317=ORIENTED_EDGE('',*,*,#9789,.T.);
#14318=ORIENTED_EDGE('',*,*,#9790,.T.);
#14319=ORIENTED_EDGE('',*,*,#9791,.T.);
#14320=ORIENTED_EDGE('',*,*,#9792,.T.);
#14321=ORIENTED_EDGE('',*,*,#9787,.T.);
#14322=ORIENTED_EDGE('',*,*,#9782,.T.);
#14323=ORIENTED_EDGE('',*,*,#9788,.F.);
#14324=ORIENTED_EDGE('',*,*,#9792,.F.);
#14325=ORIENTED_EDGE('',*,*,#9793,.T.);
#14326=ORIENTED_EDGE('',*,*,#9794,.F.);
#14327=ORIENTED_EDGE('',*,*,#9752,.F.);
#14328=ORIENTED_EDGE('',*,*,#9756,.F.);
#14329=ORIENTED_EDGE('',*,*,#9759,.F.);
#14330=ORIENTED_EDGE('',*,*,#9762,.F.);
#14331=ORIENTED_EDGE('',*,*,#9765,.F.);
#14332=ORIENTED_EDGE('',*,*,#9768,.F.);
#14333=ORIENTED_EDGE('',*,*,#9771,.F.);
#14334=ORIENTED_EDGE('',*,*,#9774,.F.);
#14335=ORIENTED_EDGE('',*,*,#9777,.F.);
#14336=ORIENTED_EDGE('',*,*,#9780,.F.);
#14337=ORIENTED_EDGE('',*,*,#9783,.F.);
#14338=ORIENTED_EDGE('',*,*,#9793,.F.);
#14339=ORIENTED_EDGE('',*,*,#9791,.F.);
#14340=ORIENTED_EDGE('',*,*,#9718,.F.);
#14341=ORIENTED_EDGE('',*,*,#9722,.F.);
#14342=ORIENTED_EDGE('',*,*,#9725,.F.);
#14343=ORIENTED_EDGE('',*,*,#9728,.F.);
#14344=ORIENTED_EDGE('',*,*,#9731,.F.);
#14345=ORIENTED_EDGE('',*,*,#9734,.F.);
#14346=ORIENTED_EDGE('',*,*,#9737,.F.);
#14347=ORIENTED_EDGE('',*,*,#9740,.F.);
#14348=ORIENTED_EDGE('',*,*,#9743,.F.);
#14349=ORIENTED_EDGE('',*,*,#9746,.F.);
#14350=ORIENTED_EDGE('',*,*,#9749,.F.);
#14351=ORIENTED_EDGE('',*,*,#9795,.F.);
#14352=ORIENTED_EDGE('',*,*,#9796,.F.);
#14353=ORIENTED_EDGE('',*,*,#9797,.T.);
#14354=ORIENTED_EDGE('',*,*,#9798,.F.);
#14355=ORIENTED_EDGE('',*,*,#9799,.F.);
#14356=ORIENTED_EDGE('',*,*,#9800,.F.);
#14357=ORIENTED_EDGE('',*,*,#9801,.F.);
#14358=ORIENTED_EDGE('',*,*,#9802,.F.);
#14359=ORIENTED_EDGE('',*,*,#9797,.F.);
#14360=ORIENTED_EDGE('',*,*,#9803,.F.);
#14361=ORIENTED_EDGE('',*,*,#9804,.T.);
#14362=ORIENTED_EDGE('',*,*,#9805,.F.);
#14363=ORIENTED_EDGE('',*,*,#9806,.F.);
#14364=ORIENTED_EDGE('',*,*,#9807,.F.);
#14365=ORIENTED_EDGE('',*,*,#9808,.F.);
#14366=ORIENTED_EDGE('',*,*,#9809,.F.);
#14367=ORIENTED_EDGE('',*,*,#9804,.F.);
#14368=ORIENTED_EDGE('',*,*,#9810,.F.);
#14369=ORIENTED_EDGE('',*,*,#9811,.T.);
#14370=ORIENTED_EDGE('',*,*,#9812,.F.);
#14371=ORIENTED_EDGE('',*,*,#9813,.F.);
#14372=ORIENTED_EDGE('',*,*,#9814,.F.);
#14373=ORIENTED_EDGE('',*,*,#9815,.F.);
#14374=ORIENTED_EDGE('',*,*,#9816,.F.);
#14375=ORIENTED_EDGE('',*,*,#9811,.F.);
#14376=ORIENTED_EDGE('',*,*,#9817,.F.);
#14377=ORIENTED_EDGE('',*,*,#9818,.T.);
#14378=ORIENTED_EDGE('',*,*,#9819,.F.);
#14379=ORIENTED_EDGE('',*,*,#9820,.F.);
#14380=ORIENTED_EDGE('',*,*,#9821,.F.);
#14381=ORIENTED_EDGE('',*,*,#9822,.F.);
#14382=ORIENTED_EDGE('',*,*,#9823,.F.);
#14383=ORIENTED_EDGE('',*,*,#9818,.F.);
#14384=ORIENTED_EDGE('',*,*,#9824,.F.);
#14385=ORIENTED_EDGE('',*,*,#9825,.T.);
#14386=ORIENTED_EDGE('',*,*,#9826,.F.);
#14387=ORIENTED_EDGE('',*,*,#9827,.F.);
#14388=ORIENTED_EDGE('',*,*,#9828,.F.);
#14389=ORIENTED_EDGE('',*,*,#9829,.F.);
#14390=ORIENTED_EDGE('',*,*,#9830,.F.);
#14391=ORIENTED_EDGE('',*,*,#9825,.F.);
#14392=ORIENTED_EDGE('',*,*,#9831,.F.);
#14393=ORIENTED_EDGE('',*,*,#9832,.T.);
#14394=ORIENTED_EDGE('',*,*,#9833,.F.);
#14395=ORIENTED_EDGE('',*,*,#9834,.F.);
#14396=ORIENTED_EDGE('',*,*,#9835,.F.);
#14397=ORIENTED_EDGE('',*,*,#9836,.F.);
#14398=ORIENTED_EDGE('',*,*,#9837,.F.);
#14399=ORIENTED_EDGE('',*,*,#9832,.F.);
#14400=ORIENTED_EDGE('',*,*,#9838,.F.);
#14401=ORIENTED_EDGE('',*,*,#9839,.T.);
#14402=ORIENTED_EDGE('',*,*,#9840,.F.);
#14403=ORIENTED_EDGE('',*,*,#9841,.F.);
#14404=ORIENTED_EDGE('',*,*,#9842,.F.);
#14405=ORIENTED_EDGE('',*,*,#9843,.F.);
#14406=ORIENTED_EDGE('',*,*,#9844,.F.);
#14407=ORIENTED_EDGE('',*,*,#9839,.F.);
#14408=ORIENTED_EDGE('',*,*,#9845,.F.);
#14409=ORIENTED_EDGE('',*,*,#9846,.T.);
#14410=ORIENTED_EDGE('',*,*,#9847,.F.);
#14411=ORIENTED_EDGE('',*,*,#9848,.F.);
#14412=ORIENTED_EDGE('',*,*,#9849,.F.);
#14413=ORIENTED_EDGE('',*,*,#9850,.F.);
#14414=ORIENTED_EDGE('',*,*,#9851,.F.);
#14415=ORIENTED_EDGE('',*,*,#9846,.F.);
#14416=ORIENTED_EDGE('',*,*,#9852,.F.);
#14417=ORIENTED_EDGE('',*,*,#9853,.T.);
#14418=ORIENTED_EDGE('',*,*,#9854,.F.);
#14419=ORIENTED_EDGE('',*,*,#9855,.F.);
#14420=ORIENTED_EDGE('',*,*,#9856,.F.);
#14421=ORIENTED_EDGE('',*,*,#9857,.F.);
#14422=ORIENTED_EDGE('',*,*,#9858,.F.);
#14423=ORIENTED_EDGE('',*,*,#9853,.F.);
#14424=ORIENTED_EDGE('',*,*,#9859,.F.);
#14425=ORIENTED_EDGE('',*,*,#9860,.T.);
#14426=ORIENTED_EDGE('',*,*,#9861,.F.);
#14427=ORIENTED_EDGE('',*,*,#9862,.F.);
#14428=ORIENTED_EDGE('',*,*,#9863,.F.);
#14429=ORIENTED_EDGE('',*,*,#9864,.F.);
#14430=ORIENTED_EDGE('',*,*,#9865,.F.);
#14431=ORIENTED_EDGE('',*,*,#9860,.F.);
#14432=ORIENTED_EDGE('',*,*,#9866,.F.);
#14433=ORIENTED_EDGE('',*,*,#9867,.T.);
#14434=ORIENTED_EDGE('',*,*,#9868,.F.);
#14435=ORIENTED_EDGE('',*,*,#9869,.F.);
#14436=ORIENTED_EDGE('',*,*,#9870,.F.);
#14437=ORIENTED_EDGE('',*,*,#9871,.F.);
#14438=ORIENTED_EDGE('',*,*,#9872,.F.);
#14439=ORIENTED_EDGE('',*,*,#9867,.F.);
#14440=ORIENTED_EDGE('',*,*,#9873,.F.);
#14441=ORIENTED_EDGE('',*,*,#9874,.T.);
#14442=ORIENTED_EDGE('',*,*,#9875,.F.);
#14443=ORIENTED_EDGE('',*,*,#9876,.F.);
#14444=ORIENTED_EDGE('',*,*,#9877,.F.);
#14445=ORIENTED_EDGE('',*,*,#9878,.F.);
#14446=ORIENTED_EDGE('',*,*,#9879,.F.);
#14447=ORIENTED_EDGE('',*,*,#9874,.F.);
#14448=ORIENTED_EDGE('',*,*,#9880,.F.);
#14449=ORIENTED_EDGE('',*,*,#9881,.T.);
#14450=ORIENTED_EDGE('',*,*,#9882,.F.);
#14451=ORIENTED_EDGE('',*,*,#9883,.F.);
#14452=ORIENTED_EDGE('',*,*,#9884,.F.);
#14453=ORIENTED_EDGE('',*,*,#9885,.F.);
#14454=ORIENTED_EDGE('',*,*,#9886,.F.);
#14455=ORIENTED_EDGE('',*,*,#9881,.F.);
#14456=ORIENTED_EDGE('',*,*,#9887,.F.);
#14457=ORIENTED_EDGE('',*,*,#9888,.T.);
#14458=ORIENTED_EDGE('',*,*,#9889,.F.);
#14459=ORIENTED_EDGE('',*,*,#9890,.F.);
#14460=ORIENTED_EDGE('',*,*,#9891,.F.);
#14461=ORIENTED_EDGE('',*,*,#9892,.F.);
#14462=ORIENTED_EDGE('',*,*,#9893,.F.);
#14463=ORIENTED_EDGE('',*,*,#9888,.F.);
#14464=ORIENTED_EDGE('',*,*,#9894,.F.);
#14465=ORIENTED_EDGE('',*,*,#9895,.T.);
#14466=ORIENTED_EDGE('',*,*,#9896,.F.);
#14467=ORIENTED_EDGE('',*,*,#9897,.F.);
#14468=ORIENTED_EDGE('',*,*,#9898,.F.);
#14469=ORIENTED_EDGE('',*,*,#9899,.F.);
#14470=ORIENTED_EDGE('',*,*,#9900,.F.);
#14471=ORIENTED_EDGE('',*,*,#9895,.F.);
#14472=ORIENTED_EDGE('',*,*,#9901,.F.);
#14473=ORIENTED_EDGE('',*,*,#9902,.T.);
#14474=ORIENTED_EDGE('',*,*,#9903,.F.);
#14475=ORIENTED_EDGE('',*,*,#9904,.F.);
#14476=ORIENTED_EDGE('',*,*,#9905,.F.);
#14477=ORIENTED_EDGE('',*,*,#9906,.F.);
#14478=ORIENTED_EDGE('',*,*,#9907,.F.);
#14479=ORIENTED_EDGE('',*,*,#9902,.F.);
#14480=ORIENTED_EDGE('',*,*,#9908,.F.);
#14481=ORIENTED_EDGE('',*,*,#9909,.T.);
#14482=ORIENTED_EDGE('',*,*,#9910,.F.);
#14483=ORIENTED_EDGE('',*,*,#9911,.F.);
#14484=ORIENTED_EDGE('',*,*,#9912,.F.);
#14485=ORIENTED_EDGE('',*,*,#9913,.F.);
#14486=ORIENTED_EDGE('',*,*,#9914,.F.);
#14487=ORIENTED_EDGE('',*,*,#9909,.F.);
#14488=ORIENTED_EDGE('',*,*,#9915,.F.);
#14489=ORIENTED_EDGE('',*,*,#9916,.T.);
#14490=ORIENTED_EDGE('',*,*,#9917,.F.);
#14491=ORIENTED_EDGE('',*,*,#9918,.F.);
#14492=ORIENTED_EDGE('',*,*,#9919,.F.);
#14493=ORIENTED_EDGE('',*,*,#9920,.F.);
#14494=ORIENTED_EDGE('',*,*,#9921,.F.);
#14495=ORIENTED_EDGE('',*,*,#9916,.F.);
#14496=ORIENTED_EDGE('',*,*,#9922,.F.);
#14497=ORIENTED_EDGE('',*,*,#9923,.T.);
#14498=ORIENTED_EDGE('',*,*,#9924,.F.);
#14499=ORIENTED_EDGE('',*,*,#9925,.F.);
#14500=ORIENTED_EDGE('',*,*,#9926,.F.);
#14501=ORIENTED_EDGE('',*,*,#9927,.F.);
#14502=ORIENTED_EDGE('',*,*,#9928,.F.);
#14503=ORIENTED_EDGE('',*,*,#9923,.F.);
#14504=ORIENTED_EDGE('',*,*,#9929,.F.);
#14505=ORIENTED_EDGE('',*,*,#9930,.T.);
#14506=ORIENTED_EDGE('',*,*,#9931,.F.);
#14507=ORIENTED_EDGE('',*,*,#9932,.F.);
#14508=ORIENTED_EDGE('',*,*,#9933,.F.);
#14509=ORIENTED_EDGE('',*,*,#9934,.F.);
#14510=ORIENTED_EDGE('',*,*,#9935,.F.);
#14511=ORIENTED_EDGE('',*,*,#9930,.F.);
#14512=ORIENTED_EDGE('',*,*,#9936,.F.);
#14513=ORIENTED_EDGE('',*,*,#9937,.T.);
#14514=ORIENTED_EDGE('',*,*,#9938,.F.);
#14515=ORIENTED_EDGE('',*,*,#9939,.F.);
#14516=ORIENTED_EDGE('',*,*,#9940,.F.);
#14517=ORIENTED_EDGE('',*,*,#9941,.F.);
#14518=ORIENTED_EDGE('',*,*,#9942,.F.);
#14519=ORIENTED_EDGE('',*,*,#9937,.F.);
#14520=ORIENTED_EDGE('',*,*,#9943,.F.);
#14521=ORIENTED_EDGE('',*,*,#9944,.T.);
#14522=ORIENTED_EDGE('',*,*,#9945,.F.);
#14523=ORIENTED_EDGE('',*,*,#9946,.F.);
#14524=ORIENTED_EDGE('',*,*,#9947,.F.);
#14525=ORIENTED_EDGE('',*,*,#9948,.F.);
#14526=ORIENTED_EDGE('',*,*,#9949,.F.);
#14527=ORIENTED_EDGE('',*,*,#9944,.F.);
#14528=ORIENTED_EDGE('',*,*,#9950,.F.);
#14529=ORIENTED_EDGE('',*,*,#9951,.T.);
#14530=ORIENTED_EDGE('',*,*,#9952,.F.);
#14531=ORIENTED_EDGE('',*,*,#9953,.F.);
#14532=ORIENTED_EDGE('',*,*,#9954,.F.);
#14533=ORIENTED_EDGE('',*,*,#9955,.F.);
#14534=ORIENTED_EDGE('',*,*,#9956,.F.);
#14535=ORIENTED_EDGE('',*,*,#9951,.F.);
#14536=ORIENTED_EDGE('',*,*,#9957,.F.);
#14537=ORIENTED_EDGE('',*,*,#9958,.T.);
#14538=ORIENTED_EDGE('',*,*,#9959,.F.);
#14539=ORIENTED_EDGE('',*,*,#9960,.F.);
#14540=ORIENTED_EDGE('',*,*,#9961,.F.);
#14541=ORIENTED_EDGE('',*,*,#9962,.F.);
#14542=ORIENTED_EDGE('',*,*,#9963,.F.);
#14543=ORIENTED_EDGE('',*,*,#9958,.F.);
#14544=ORIENTED_EDGE('',*,*,#9920,.T.);
#14545=ORIENTED_EDGE('',*,*,#9964,.F.);
#14546=ORIENTED_EDGE('',*,*,#9960,.T.);
#14547=ORIENTED_EDGE('',*,*,#9965,.T.);
#14548=ORIENTED_EDGE('',*,*,#9878,.T.);
#14549=ORIENTED_EDGE('',*,*,#9966,.F.);
#14550=ORIENTED_EDGE('',*,*,#9918,.T.);
#14551=ORIENTED_EDGE('',*,*,#9967,.T.);
#14552=ORIENTED_EDGE('',*,*,#9876,.T.);
#14553=ORIENTED_EDGE('',*,*,#9968,.T.);
#14554=ORIENTED_EDGE('',*,*,#9885,.T.);
#14555=ORIENTED_EDGE('',*,*,#9969,.F.);
#14556=ORIENTED_EDGE('',*,*,#9871,.T.);
#14557=ORIENTED_EDGE('',*,*,#9970,.F.);
#14558=ORIENTED_EDGE('',*,*,#9883,.T.);
#14559=ORIENTED_EDGE('',*,*,#9971,.T.);
#14560=ORIENTED_EDGE('',*,*,#9869,.T.);
#14561=ORIENTED_EDGE('',*,*,#9972,.T.);
#14562=ORIENTED_EDGE('',*,*,#9892,.T.);
#14563=ORIENTED_EDGE('',*,*,#9973,.F.);
#14564=ORIENTED_EDGE('',*,*,#9864,.T.);
#14565=ORIENTED_EDGE('',*,*,#9974,.F.);
#14566=ORIENTED_EDGE('',*,*,#9890,.T.);
#14567=ORIENTED_EDGE('',*,*,#9975,.T.);
#14568=ORIENTED_EDGE('',*,*,#9862,.T.);
#14569=ORIENTED_EDGE('',*,*,#9976,.T.);
#14570=ORIENTED_EDGE('',*,*,#9899,.T.);
#14571=ORIENTED_EDGE('',*,*,#9977,.F.);
#14572=ORIENTED_EDGE('',*,*,#9857,.T.);
#14573=ORIENTED_EDGE('',*,*,#9978,.F.);
#14574=ORIENTED_EDGE('',*,*,#9897,.T.);
#14575=ORIENTED_EDGE('',*,*,#9979,.T.);
#14576=ORIENTED_EDGE('',*,*,#9855,.T.);
#14577=ORIENTED_EDGE('',*,*,#9980,.T.);
#14578=ORIENTED_EDGE('',*,*,#9906,.T.);
#14579=ORIENTED_EDGE('',*,*,#9981,.F.);
#14580=ORIENTED_EDGE('',*,*,#9850,.T.);
#14581=ORIENTED_EDGE('',*,*,#9982,.F.);
#14582=ORIENTED_EDGE('',*,*,#9904,.T.);
#14583=ORIENTED_EDGE('',*,*,#9983,.T.);
#14584=ORIENTED_EDGE('',*,*,#9848,.T.);
#14585=ORIENTED_EDGE('',*,*,#9984,.T.);
#14586=ORIENTED_EDGE('',*,*,#9913,.T.);
#14587=ORIENTED_EDGE('',*,*,#9985,.F.);
#14588=ORIENTED_EDGE('',*,*,#9843,.T.);
#14589=ORIENTED_EDGE('',*,*,#9986,.F.);
#14590=ORIENTED_EDGE('',*,*,#9911,.T.);
#14591=ORIENTED_EDGE('',*,*,#9987,.T.);
#14592=ORIENTED_EDGE('',*,*,#9836,.T.);
#14593=ORIENTED_EDGE('',*,*,#9988,.F.);
#14594=ORIENTED_EDGE('',*,*,#9841,.T.);
#14595=ORIENTED_EDGE('',*,*,#9989,.T.);
#14596=ORIENTED_EDGE('',*,*,#9834,.T.);
#14597=ORIENTED_EDGE('',*,*,#9990,.T.);
#14598=ORIENTED_EDGE('',*,*,#9927,.T.);
#14599=ORIENTED_EDGE('',*,*,#9991,.F.);
#14600=ORIENTED_EDGE('',*,*,#9829,.T.);
#14601=ORIENTED_EDGE('',*,*,#9992,.F.);
#14602=ORIENTED_EDGE('',*,*,#9925,.T.);
#14603=ORIENTED_EDGE('',*,*,#9993,.T.);
#14604=ORIENTED_EDGE('',*,*,#9827,.T.);
#14605=ORIENTED_EDGE('',*,*,#9994,.T.);
#14606=ORIENTED_EDGE('',*,*,#9934,.T.);
#14607=ORIENTED_EDGE('',*,*,#9995,.F.);
#14608=ORIENTED_EDGE('',*,*,#9822,.T.);
#14609=ORIENTED_EDGE('',*,*,#9996,.F.);
#14610=ORIENTED_EDGE('',*,*,#9932,.T.);
#14611=ORIENTED_EDGE('',*,*,#9997,.T.);
#14612=ORIENTED_EDGE('',*,*,#9820,.T.);
#14613=ORIENTED_EDGE('',*,*,#9998,.T.);
#14614=ORIENTED_EDGE('',*,*,#9941,.T.);
#14615=ORIENTED_EDGE('',*,*,#9999,.F.);
#14616=ORIENTED_EDGE('',*,*,#9815,.T.);
#14617=ORIENTED_EDGE('',*,*,#10000,.F.);
#14618=ORIENTED_EDGE('',*,*,#9939,.T.);
#14619=ORIENTED_EDGE('',*,*,#10001,.T.);
#14620=ORIENTED_EDGE('',*,*,#9813,.T.);
#14621=ORIENTED_EDGE('',*,*,#10002,.T.);
#14622=ORIENTED_EDGE('',*,*,#9948,.T.);
#14623=ORIENTED_EDGE('',*,*,#10003,.F.);
#14624=ORIENTED_EDGE('',*,*,#9808,.T.);
#14625=ORIENTED_EDGE('',*,*,#10004,.F.);
#14626=ORIENTED_EDGE('',*,*,#9946,.T.);
#14627=ORIENTED_EDGE('',*,*,#10005,.T.);
#14628=ORIENTED_EDGE('',*,*,#9806,.T.);
#14629=ORIENTED_EDGE('',*,*,#10006,.T.);
#14630=ORIENTED_EDGE('',*,*,#9955,.T.);
#14631=ORIENTED_EDGE('',*,*,#10007,.F.);
#14632=ORIENTED_EDGE('',*,*,#9801,.T.);
#14633=ORIENTED_EDGE('',*,*,#10008,.F.);
#14634=ORIENTED_EDGE('',*,*,#9953,.T.);
#14635=ORIENTED_EDGE('',*,*,#10009,.T.);
#14636=ORIENTED_EDGE('',*,*,#9799,.T.);
#14637=ORIENTED_EDGE('',*,*,#10010,.T.);
#14638=ORIENTED_EDGE('',*,*,#9962,.T.);
#14639=ORIENTED_EDGE('',*,*,#10011,.F.);
#14640=ORIENTED_EDGE('',*,*,#9798,.T.);
#14641=ORIENTED_EDGE('',*,*,#9802,.T.);
#14642=ORIENTED_EDGE('',*,*,#10009,.F.);
#14643=ORIENTED_EDGE('',*,*,#9952,.T.);
#14644=ORIENTED_EDGE('',*,*,#9956,.T.);
#14645=ORIENTED_EDGE('',*,*,#10006,.F.);
#14646=ORIENTED_EDGE('',*,*,#9805,.T.);
#14647=ORIENTED_EDGE('',*,*,#9809,.T.);
#14648=ORIENTED_EDGE('',*,*,#10005,.F.);
#14649=ORIENTED_EDGE('',*,*,#9945,.T.);
#14650=ORIENTED_EDGE('',*,*,#9949,.T.);
#14651=ORIENTED_EDGE('',*,*,#10002,.F.);
#14652=ORIENTED_EDGE('',*,*,#9812,.T.);
#14653=ORIENTED_EDGE('',*,*,#9816,.T.);
#14654=ORIENTED_EDGE('',*,*,#10001,.F.);
#14655=ORIENTED_EDGE('',*,*,#9938,.T.);
#14656=ORIENTED_EDGE('',*,*,#9942,.T.);
#14657=ORIENTED_EDGE('',*,*,#9998,.F.);
#14658=ORIENTED_EDGE('',*,*,#9819,.T.);
#14659=ORIENTED_EDGE('',*,*,#9823,.T.);
#14660=ORIENTED_EDGE('',*,*,#9997,.F.);
#14661=ORIENTED_EDGE('',*,*,#9931,.T.);
#14662=ORIENTED_EDGE('',*,*,#9935,.T.);
#14663=ORIENTED_EDGE('',*,*,#9994,.F.);
#14664=ORIENTED_EDGE('',*,*,#9826,.T.);
#14665=ORIENTED_EDGE('',*,*,#9830,.T.);
#14666=ORIENTED_EDGE('',*,*,#9993,.F.);
#14667=ORIENTED_EDGE('',*,*,#9924,.T.);
#14668=ORIENTED_EDGE('',*,*,#9928,.T.);
#14669=ORIENTED_EDGE('',*,*,#9990,.F.);
#14670=ORIENTED_EDGE('',*,*,#9833,.T.);
#14671=ORIENTED_EDGE('',*,*,#10012,.T.);
#14672=ORIENTED_EDGE('',*,*,#10013,.T.);
#14673=ORIENTED_EDGE('',*,*,#10012,.F.);
#14674=ORIENTED_EDGE('',*,*,#9837,.T.);
#14675=ORIENTED_EDGE('',*,*,#9989,.F.);
#14676=ORIENTED_EDGE('',*,*,#9840,.T.);
#14677=ORIENTED_EDGE('',*,*,#9844,.T.);
#14678=ORIENTED_EDGE('',*,*,#9987,.F.);
#14679=ORIENTED_EDGE('',*,*,#9910,.T.);
#14680=ORIENTED_EDGE('',*,*,#9914,.T.);
#14681=ORIENTED_EDGE('',*,*,#9984,.F.);
#14682=ORIENTED_EDGE('',*,*,#9847,.T.);
#14683=ORIENTED_EDGE('',*,*,#9851,.T.);
#14684=ORIENTED_EDGE('',*,*,#9983,.F.);
#14685=ORIENTED_EDGE('',*,*,#9903,.T.);
#14686=ORIENTED_EDGE('',*,*,#9907,.T.);
#14687=ORIENTED_EDGE('',*,*,#9980,.F.);
#14688=ORIENTED_EDGE('',*,*,#9854,.T.);
#14689=ORIENTED_EDGE('',*,*,#9858,.T.);
#14690=ORIENTED_EDGE('',*,*,#9979,.F.);
#14691=ORIENTED_EDGE('',*,*,#9896,.T.);
#14692=ORIENTED_EDGE('',*,*,#9900,.T.);
#14693=ORIENTED_EDGE('',*,*,#9976,.F.);
#14694=ORIENTED_EDGE('',*,*,#9861,.T.);
#14695=ORIENTED_EDGE('',*,*,#9865,.T.);
#14696=ORIENTED_EDGE('',*,*,#9975,.F.);
#14697=ORIENTED_EDGE('',*,*,#9889,.T.);
#14698=ORIENTED_EDGE('',*,*,#9893,.T.);
#14699=ORIENTED_EDGE('',*,*,#9972,.F.);
#14700=ORIENTED_EDGE('',*,*,#9868,.T.);
#14701=ORIENTED_EDGE('',*,*,#9872,.T.);
#14702=ORIENTED_EDGE('',*,*,#9971,.F.);
#14703=ORIENTED_EDGE('',*,*,#9882,.T.);
#14704=ORIENTED_EDGE('',*,*,#9886,.T.);
#14705=ORIENTED_EDGE('',*,*,#9968,.F.);
#14706=ORIENTED_EDGE('',*,*,#9875,.T.);
#14707=ORIENTED_EDGE('',*,*,#9879,.T.);
#14708=ORIENTED_EDGE('',*,*,#9967,.F.);
#14709=ORIENTED_EDGE('',*,*,#9917,.T.);
#14710=ORIENTED_EDGE('',*,*,#9921,.T.);
#14711=ORIENTED_EDGE('',*,*,#9965,.F.);
#14712=ORIENTED_EDGE('',*,*,#9959,.T.);
#14713=ORIENTED_EDGE('',*,*,#9963,.T.);
#14714=ORIENTED_EDGE('',*,*,#10010,.F.);
#14715=ORIENTED_EDGE('',*,*,#10014,.F.);
#14716=ORIENTED_EDGE('',*,*,#9789,.F.);
#14717=ORIENTED_EDGE('',*,*,#9719,.F.);
#14718=ORIENTED_EDGE('',*,*,#9790,.F.);
#14719=ORIENTED_EDGE('',*,*,#10015,.T.);
#14720=ORIENTED_EDGE('',*,*,#10014,.T.);
#14721=ORIENTED_EDGE('',*,*,#10015,.F.);
#14722=ORIENTED_EDGE('',*,*,#9748,.T.);
#14723=ORIENTED_EDGE('',*,*,#9786,.T.);
#14724=ORIENTED_EDGE('',*,*,#10016,.F.);
#14725=ORIENTED_EDGE('',*,*,#9795,.T.);
#14726=ORIENTED_EDGE('',*,*,#10013,.F.);
#14727=ORIENTED_EDGE('',*,*,#10016,.T.);
#14728=ORIENTED_EDGE('',*,*,#9785,.T.);
#14729=ORIENTED_EDGE('',*,*,#9753,.T.);
#14730=ORIENTED_EDGE('',*,*,#9794,.T.);
#14731=ORIENTED_EDGE('',*,*,#10017,.F.);
#14732=ORIENTED_EDGE('',*,*,#10018,.T.);
#14733=ORIENTED_EDGE('',*,*,#9831,.T.);
#14734=ORIENTED_EDGE('',*,*,#9991,.T.);
#14735=ORIENTED_EDGE('',*,*,#9926,.T.);
#14736=ORIENTED_EDGE('',*,*,#9922,.T.);
#14737=ORIENTED_EDGE('',*,*,#9992,.T.);
#14738=ORIENTED_EDGE('',*,*,#9828,.T.);
#14739=ORIENTED_EDGE('',*,*,#9824,.T.);
#14740=ORIENTED_EDGE('',*,*,#9995,.T.);
#14741=ORIENTED_EDGE('',*,*,#9933,.T.);
#14742=ORIENTED_EDGE('',*,*,#9929,.T.);
#14743=ORIENTED_EDGE('',*,*,#9996,.T.);
#14744=ORIENTED_EDGE('',*,*,#9821,.T.);
#14745=ORIENTED_EDGE('',*,*,#9817,.T.);
#14746=ORIENTED_EDGE('',*,*,#9999,.T.);
#14747=ORIENTED_EDGE('',*,*,#9940,.T.);
#14748=ORIENTED_EDGE('',*,*,#9936,.T.);
#14749=ORIENTED_EDGE('',*,*,#10000,.T.);
#14750=ORIENTED_EDGE('',*,*,#9814,.T.);
#14751=ORIENTED_EDGE('',*,*,#9810,.T.);
#14752=ORIENTED_EDGE('',*,*,#10003,.T.);
#14753=ORIENTED_EDGE('',*,*,#9947,.T.);
#14754=ORIENTED_EDGE('',*,*,#9943,.T.);
#14755=ORIENTED_EDGE('',*,*,#10004,.T.);
#14756=ORIENTED_EDGE('',*,*,#9807,.T.);
#14757=ORIENTED_EDGE('',*,*,#9803,.T.);
#14758=ORIENTED_EDGE('',*,*,#10007,.T.);
#14759=ORIENTED_EDGE('',*,*,#9954,.T.);
#14760=ORIENTED_EDGE('',*,*,#9950,.T.);
#14761=ORIENTED_EDGE('',*,*,#10008,.T.);
#14762=ORIENTED_EDGE('',*,*,#9800,.T.);
#14763=ORIENTED_EDGE('',*,*,#9796,.T.);
#14764=ORIENTED_EDGE('',*,*,#10011,.T.);
#14765=ORIENTED_EDGE('',*,*,#9961,.T.);
#14766=ORIENTED_EDGE('',*,*,#9957,.T.);
#14767=ORIENTED_EDGE('',*,*,#9964,.T.);
#14768=ORIENTED_EDGE('',*,*,#9919,.T.);
#14769=ORIENTED_EDGE('',*,*,#9915,.T.);
#14770=ORIENTED_EDGE('',*,*,#9966,.T.);
#14771=ORIENTED_EDGE('',*,*,#9877,.T.);
#14772=ORIENTED_EDGE('',*,*,#9873,.T.);
#14773=ORIENTED_EDGE('',*,*,#9969,.T.);
#14774=ORIENTED_EDGE('',*,*,#9884,.T.);
#14775=ORIENTED_EDGE('',*,*,#9880,.T.);
#14776=ORIENTED_EDGE('',*,*,#9970,.T.);
#14777=ORIENTED_EDGE('',*,*,#9870,.T.);
#14778=ORIENTED_EDGE('',*,*,#9866,.T.);
#14779=ORIENTED_EDGE('',*,*,#9973,.T.);
#14780=ORIENTED_EDGE('',*,*,#9891,.T.);
#14781=ORIENTED_EDGE('',*,*,#9887,.T.);
#14782=ORIENTED_EDGE('',*,*,#9974,.T.);
#14783=ORIENTED_EDGE('',*,*,#9863,.T.);
#14784=ORIENTED_EDGE('',*,*,#9859,.T.);
#14785=ORIENTED_EDGE('',*,*,#9977,.T.);
#14786=ORIENTED_EDGE('',*,*,#9898,.T.);
#14787=ORIENTED_EDGE('',*,*,#9894,.T.);
#14788=ORIENTED_EDGE('',*,*,#9978,.T.);
#14789=ORIENTED_EDGE('',*,*,#9856,.T.);
#14790=ORIENTED_EDGE('',*,*,#9852,.T.);
#14791=ORIENTED_EDGE('',*,*,#9981,.T.);
#14792=ORIENTED_EDGE('',*,*,#9905,.T.);
#14793=ORIENTED_EDGE('',*,*,#9901,.T.);
#14794=ORIENTED_EDGE('',*,*,#9982,.T.);
#14795=ORIENTED_EDGE('',*,*,#9849,.T.);
#14796=ORIENTED_EDGE('',*,*,#9845,.T.);
#14797=ORIENTED_EDGE('',*,*,#9985,.T.);
#14798=ORIENTED_EDGE('',*,*,#9912,.T.);
#14799=ORIENTED_EDGE('',*,*,#9908,.T.);
#14800=ORIENTED_EDGE('',*,*,#9986,.T.);
#14801=ORIENTED_EDGE('',*,*,#9842,.T.);
#14802=ORIENTED_EDGE('',*,*,#9838,.T.);
#14803=ORIENTED_EDGE('',*,*,#9988,.T.);
#14804=ORIENTED_EDGE('',*,*,#9835,.T.);
#14805=ORIENTED_EDGE('',*,*,#10018,.F.);
#14806=ORIENTED_EDGE('',*,*,#10017,.T.);
#15265=PLANE('',#17648);
#15266=PLANE('',#17653);
#15267=PLANE('',#17654);
#15268=PLANE('',#17655);
#15269=PLANE('',#17656);
#15270=PLANE('',#17657);
#15271=PLANE('',#17658);
#15272=PLANE('',#17659);
#15273=PLANE('',#17660);
#15274=PLANE('',#17661);
#15275=PLANE('',#17662);
#15276=PLANE('',#17663);
#15277=PLANE('',#17664);
#15278=PLANE('',#17665);
#15279=PLANE('',#17666);
#15280=PLANE('',#17667);
#15281=PLANE('',#17668);
#15282=PLANE('',#17669);
#15283=PLANE('',#17670);
#15284=PLANE('',#17671);
#15285=PLANE('',#17672);
#15286=PLANE('',#17673);
#15287=PLANE('',#17674);
#15288=PLANE('',#17675);
#15289=PLANE('',#17676);
#15290=PLANE('',#17677);
#15291=PLANE('',#17678);
#15292=PLANE('',#17679);
#15293=PLANE('',#17680);
#15294=PLANE('',#17681);
#15295=PLANE('',#17682);
#15296=PLANE('',#17683);
#15297=PLANE('',#17684);
#15298=PLANE('',#17685);
#15299=PLANE('',#17686);
#15300=PLANE('',#17687);
#15301=PLANE('',#17688);
#15302=PLANE('',#17689);
#15303=PLANE('',#17690);
#15304=PLANE('',#17691);
#15305=PLANE('',#17692);
#15306=PLANE('',#17693);
#15307=PLANE('',#17694);
#15308=PLANE('',#17695);
#15309=PLANE('',#17696);
#15310=PLANE('',#17697);
#15311=PLANE('',#17698);
#15312=PLANE('',#17699);
#15313=PLANE('',#17700);
#15314=PLANE('',#17775);
#15315=PLANE('',#17780);
#15316=PLANE('',#17783);
#16129=ADVANCED_FACE('',(#2586),#1111,.T.);
#16130=ADVANCED_FACE('',(#2587),#1112,.T.);
#16131=ADVANCED_FACE('',(#2588),#1113,.T.);
#16132=ADVANCED_FACE('',(#2589),#1114,.T.);
#16133=ADVANCED_FACE('',(#2590),#1115,.T.);
#16134=ADVANCED_FACE('',(#2591),#1116,.T.);
#16135=ADVANCED_FACE('',(#2592),#1117,.T.);
#16136=ADVANCED_FACE('',(#2593),#1118,.T.);
#16137=ADVANCED_FACE('',(#2594),#1119,.T.);
#16138=ADVANCED_FACE('',(#2595),#1120,.T.);
#16139=ADVANCED_FACE('',(#2596),#1121,.T.);
#16140=ADVANCED_FACE('',(#2597),#1122,.T.);
#16141=ADVANCED_FACE('',(#2598),#1123,.T.);
#16142=ADVANCED_FACE('',(#2599),#1124,.T.);
#16143=ADVANCED_FACE('',(#2600),#1125,.T.);
#16144=ADVANCED_FACE('',(#2601),#1126,.T.);
#16145=ADVANCED_FACE('',(#2602),#1127,.T.);
#16146=ADVANCED_FACE('',(#2603),#1128,.T.);
#16147=ADVANCED_FACE('',(#2604),#1129,.T.);
#16148=ADVANCED_FACE('',(#2605),#1130,.T.);
#16149=ADVANCED_FACE('',(#2606),#1131,.T.);
#16150=ADVANCED_FACE('',(#2607),#1132,.T.);
#16151=ADVANCED_FACE('',(#2608),#508,.F.);
#16152=ADVANCED_FACE('',(#2609),#15265,.T.);
#16153=ADVANCED_FACE('',(#2610),#1133,.T.);
#16154=ADVANCED_FACE('',(#2611),#509,.F.);
#16155=ADVANCED_FACE('',(#2612),#15266,.F.);
#16156=ADVANCED_FACE('',(#2613),#15267,.F.);
#16157=ADVANCED_FACE('',(#2614),#15268,.F.);
#16158=ADVANCED_FACE('',(#2615),#15269,.F.);
#16159=ADVANCED_FACE('',(#2616),#15270,.F.);
#16160=ADVANCED_FACE('',(#2617),#15271,.F.);
#16161=ADVANCED_FACE('',(#2618),#15272,.F.);
#16162=ADVANCED_FACE('',(#2619),#15273,.F.);
#16163=ADVANCED_FACE('',(#2620),#15274,.F.);
#16164=ADVANCED_FACE('',(#2621),#15275,.F.);
#16165=ADVANCED_FACE('',(#2622),#15276,.F.);
#16166=ADVANCED_FACE('',(#2623),#15277,.F.);
#16167=ADVANCED_FACE('',(#2624),#15278,.F.);
#16168=ADVANCED_FACE('',(#2625),#15279,.F.);
#16169=ADVANCED_FACE('',(#2626),#15280,.F.);
#16170=ADVANCED_FACE('',(#2627),#15281,.F.);
#16171=ADVANCED_FACE('',(#2628),#15282,.F.);
#16172=ADVANCED_FACE('',(#2629),#15283,.F.);
#16173=ADVANCED_FACE('',(#2630),#15284,.F.);
#16174=ADVANCED_FACE('',(#2631),#15285,.F.);
#16175=ADVANCED_FACE('',(#2632),#15286,.F.);
#16176=ADVANCED_FACE('',(#2633),#15287,.F.);
#16177=ADVANCED_FACE('',(#2634),#15288,.F.);
#16178=ADVANCED_FACE('',(#2635),#15289,.F.);
#16179=ADVANCED_FACE('',(#2636),#15290,.F.);
#16180=ADVANCED_FACE('',(#2637),#15291,.F.);
#16181=ADVANCED_FACE('',(#2638),#15292,.F.);
#16182=ADVANCED_FACE('',(#2639),#15293,.F.);
#16183=ADVANCED_FACE('',(#2640),#15294,.F.);
#16184=ADVANCED_FACE('',(#2641),#15295,.F.);
#16185=ADVANCED_FACE('',(#2642),#15296,.F.);
#16186=ADVANCED_FACE('',(#2643),#15297,.F.);
#16187=ADVANCED_FACE('',(#2644),#15298,.F.);
#16188=ADVANCED_FACE('',(#2645),#15299,.F.);
#16189=ADVANCED_FACE('',(#2646),#15300,.F.);
#16190=ADVANCED_FACE('',(#2647),#15301,.F.);
#16191=ADVANCED_FACE('',(#2648),#15302,.F.);
#16192=ADVANCED_FACE('',(#2649),#15303,.F.);
#16193=ADVANCED_FACE('',(#2650),#15304,.F.);
#16194=ADVANCED_FACE('',(#2651),#15305,.F.);
#16195=ADVANCED_FACE('',(#2652),#15306,.F.);
#16196=ADVANCED_FACE('',(#2653),#15307,.F.);
#16197=ADVANCED_FACE('',(#2654),#15308,.F.);
#16198=ADVANCED_FACE('',(#2655),#15309,.F.);
#16199=ADVANCED_FACE('',(#2656),#15310,.F.);
#16200=ADVANCED_FACE('',(#2657),#15311,.F.);
#16201=ADVANCED_FACE('',(#2658),#15312,.F.);
#16202=ADVANCED_FACE('',(#2659),#15313,.F.);
#16203=ADVANCED_FACE('',(#2660),#1134,.T.);
#16204=ADVANCED_FACE('',(#2661),#1135,.T.);
#16205=ADVANCED_FACE('',(#2662),#1136,.T.);
#16206=ADVANCED_FACE('',(#2663),#1137,.T.);
#16207=ADVANCED_FACE('',(#2664),#1138,.T.);
#16208=ADVANCED_FACE('',(#2665),#1139,.T.);
#16209=ADVANCED_FACE('',(#2666),#1140,.T.);
#16210=ADVANCED_FACE('',(#2667),#1141,.T.);
#16211=ADVANCED_FACE('',(#2668),#1142,.T.);
#16212=ADVANCED_FACE('',(#2669),#1143,.T.);
#16213=ADVANCED_FACE('',(#2670),#1144,.T.);
#16214=ADVANCED_FACE('',(#2671),#1145,.T.);
#16215=ADVANCED_FACE('',(#2672),#1146,.T.);
#16216=ADVANCED_FACE('',(#2673),#1147,.T.);
#16217=ADVANCED_FACE('',(#2674),#1148,.T.);
#16218=ADVANCED_FACE('',(#2675),#1149,.T.);
#16219=ADVANCED_FACE('',(#2676),#1150,.T.);
#16220=ADVANCED_FACE('',(#2677),#1151,.T.);
#16221=ADVANCED_FACE('',(#2678),#1152,.T.);
#16222=ADVANCED_FACE('',(#2679),#1153,.T.);
#16223=ADVANCED_FACE('',(#2680),#1154,.T.);
#16224=ADVANCED_FACE('',(#2681),#1155,.T.);
#16225=ADVANCED_FACE('',(#2682),#1156,.T.);
#16226=ADVANCED_FACE('',(#2683),#1157,.T.);
#16227=ADVANCED_FACE('',(#2684),#1771,.T.);
#16228=ADVANCED_FACE('',(#2685),#15314,.T.);
#16229=ADVANCED_FACE('',(#2686),#1772,.T.);
#16230=ADVANCED_FACE('',(#2687),#1158,.T.);
#16231=ADVANCED_FACE('',(#2688,#1204),#15315,.T.);
#16232=ADVANCED_FACE('',(#2689),#1773,.T.);
#16233=ADVANCED_FACE('',(#2690),#15316,.T.);
#16247=CLOSED_SHELL('',(#16129,#16130,#16131,#16132,#16133,#16134,#16135,
#16136,#16137,#16138,#16139,#16140,#16141,#16142,#16143,#16144,#16145,#16146,
#16147,#16148,#16149,#16150,#16151,#16152,#16153,#16154,#16155,#16156,#16157,
#16158,#16159,#16160,#16161,#16162,#16163,#16164,#16165,#16166,#16167,#16168,
#16169,#16170,#16171,#16172,#16173,#16174,#16175,#16176,#16177,#16178,#16179,
#16180,#16181,#16182,#16183,#16184,#16185,#16186,#16187,#16188,#16189,#16190,
#16191,#16192,#16193,#16194,#16195,#16196,#16197,#16198,#16199,#16200,#16201,
#16202,#16203,#16204,#16205,#16206,#16207,#16208,#16209,#16210,#16211,#16212,
#16213,#16214,#16215,#16216,#16217,#16218,#16219,#16220,#16221,#16222,#16223,
#16224,#16225,#16226,#16227,#16228,#16229,#16230,#16231,#16232,#16233));
#17623=AXIS2_PLACEMENT_3D('',#36255,#21372,#21373);
#17624=AXIS2_PLACEMENT_3D('',#36256,#21374,#21375);
#17625=AXIS2_PLACEMENT_3D('',#36272,#21377,#21378);
#17626=AXIS2_PLACEMENT_3D('',#36280,#21379,#21380);
#17627=AXIS2_PLACEMENT_3D('',#36328,#21382,#21383);
#17628=AXIS2_PLACEMENT_3D('',#36376,#21385,#21386);
#17629=AXIS2_PLACEMENT_3D('',#36430,#21388,#21389);
#17630=AXIS2_PLACEMENT_3D('',#36478,#21391,#21392);
#17631=AXIS2_PLACEMENT_3D('',#36526,#21394,#21395);
#17632=AXIS2_PLACEMENT_3D('',#36580,#21397,#21398);
#17633=AXIS2_PLACEMENT_3D('',#36628,#21400,#21401);
#17634=AXIS2_PLACEMENT_3D('',#36676,#21403,#21404);
#17635=AXIS2_PLACEMENT_3D('',#36724,#21406,#21407);
#17636=AXIS2_PLACEMENT_3D('',#36778,#21409,#21410);
#17637=AXIS2_PLACEMENT_3D('',#36790,#21412,#21413);
#17638=AXIS2_PLACEMENT_3D('',#36796,#21414,#21415);
#17639=AXIS2_PLACEMENT_3D('',#36821,#21417,#21418);
#17640=AXIS2_PLACEMENT_3D('',#36846,#21420,#21421);
#17641=AXIS2_PLACEMENT_3D('',#36870,#21423,#21424);
#17642=AXIS2_PLACEMENT_3D('',#36894,#21426,#21427);
#17643=AXIS2_PLACEMENT_3D('',#36919,#21429,#21430);
#17644=AXIS2_PLACEMENT_3D('',#36944,#21432,#21433);
#17645=AXIS2_PLACEMENT_3D('',#36968,#21435,#21436);
#17646=AXIS2_PLACEMENT_3D('',#36993,#21438,#21439);
#17647=AXIS2_PLACEMENT_3D('',#37018,#21441,#21442);
#17648=AXIS2_PLACEMENT_3D('',#37479,#21444,#21445);
#17649=AXIS2_PLACEMENT_3D('',#37481,#21446,#21447);
#17650=AXIS2_PLACEMENT_3D('',#37482,#21448,#21449);
#17651=AXIS2_PLACEMENT_3D('',#37539,#21450,#21451);
#17652=AXIS2_PLACEMENT_3D('',#37540,#21452,#21453);
#17653=AXIS2_PLACEMENT_3D('',#37918,#21454,#21455);
#17654=AXIS2_PLACEMENT_3D('',#37931,#21458,#21459);
#17655=AXIS2_PLACEMENT_3D('',#37941,#21461,#21462);
#17656=AXIS2_PLACEMENT_3D('',#37954,#21465,#21466);
#17657=AXIS2_PLACEMENT_3D('',#37964,#21468,#21469);
#17658=AXIS2_PLACEMENT_3D('',#37977,#21472,#21473);
#17659=AXIS2_PLACEMENT_3D('',#37987,#21475,#21476);
#17660=AXIS2_PLACEMENT_3D('',#38000,#21479,#21480);
#17661=AXIS2_PLACEMENT_3D('',#38010,#21482,#21483);
#17662=AXIS2_PLACEMENT_3D('',#38023,#21486,#21487);
#17663=AXIS2_PLACEMENT_3D('',#38033,#21489,#21490);
#17664=AXIS2_PLACEMENT_3D('',#38046,#21493,#21494);
#17665=AXIS2_PLACEMENT_3D('',#38056,#21496,#21497);
#17666=AXIS2_PLACEMENT_3D('',#38069,#21500,#21501);
#17667=AXIS2_PLACEMENT_3D('',#38079,#21503,#21504);
#17668=AXIS2_PLACEMENT_3D('',#38092,#21507,#21508);
#17669=AXIS2_PLACEMENT_3D('',#38102,#21510,#21511);
#17670=AXIS2_PLACEMENT_3D('',#38115,#21514,#21515);
#17671=AXIS2_PLACEMENT_3D('',#38125,#21517,#21518);
#17672=AXIS2_PLACEMENT_3D('',#38138,#21521,#21522);
#17673=AXIS2_PLACEMENT_3D('',#38148,#21524,#21525);
#17674=AXIS2_PLACEMENT_3D('',#38161,#21528,#21529);
#17675=AXIS2_PLACEMENT_3D('',#38171,#21531,#21532);
#17676=AXIS2_PLACEMENT_3D('',#38184,#21535,#21536);
#17677=AXIS2_PLACEMENT_3D('',#38194,#21538,#21539);
#17678=AXIS2_PLACEMENT_3D('',#38207,#21542,#21543);
#17679=AXIS2_PLACEMENT_3D('',#38217,#21545,#21546);
#17680=AXIS2_PLACEMENT_3D('',#38230,#21549,#21550);
#17681=AXIS2_PLACEMENT_3D('',#38240,#21552,#21553);
#17682=AXIS2_PLACEMENT_3D('',#38253,#21556,#21557);
#17683=AXIS2_PLACEMENT_3D('',#38263,#21559,#21560);
#17684=AXIS2_PLACEMENT_3D('',#38276,#21563,#21564);
#17685=AXIS2_PLACEMENT_3D('',#38286,#21566,#21567);
#17686=AXIS2_PLACEMENT_3D('',#38299,#21570,#21571);
#17687=AXIS2_PLACEMENT_3D('',#38309,#21573,#21574);
#17688=AXIS2_PLACEMENT_3D('',#38322,#21577,#21578);
#17689=AXIS2_PLACEMENT_3D('',#38332,#21580,#21581);
#17690=AXIS2_PLACEMENT_3D('',#38345,#21584,#21585);
#17691=AXIS2_PLACEMENT_3D('',#38355,#21587,#21588);
#17692=AXIS2_PLACEMENT_3D('',#38368,#21591,#21592);
#17693=AXIS2_PLACEMENT_3D('',#38378,#21594,#21595);
#17694=AXIS2_PLACEMENT_3D('',#38391,#21598,#21599);
#17695=AXIS2_PLACEMENT_3D('',#38401,#21601,#21602);
#17696=AXIS2_PLACEMENT_3D('',#38414,#21605,#21606);
#17697=AXIS2_PLACEMENT_3D('',#38424,#21608,#21609);
#17698=AXIS2_PLACEMENT_3D('',#38437,#21612,#21613);
#17699=AXIS2_PLACEMENT_3D('',#38447,#21615,#21616);
#17700=AXIS2_PLACEMENT_3D('',#38460,#21619,#21620);
#17701=AXIS2_PLACEMENT_3D('',#38470,#21622,#21623);
#17702=AXIS2_PLACEMENT_3D('',#38471,#21624,#21625);
#17703=AXIS2_PLACEMENT_3D('',#38472,#21626,#21627);
#17704=AXIS2_PLACEMENT_3D('',#38473,#21628,#21629);
#17705=AXIS2_PLACEMENT_3D('',#38474,#21630,#21631);
#17706=AXIS2_PLACEMENT_3D('',#38475,#21632,#21633);
#17707=AXIS2_PLACEMENT_3D('',#38476,#21634,#21635);
#17708=AXIS2_PLACEMENT_3D('',#38477,#21636,#21637);
#17709=AXIS2_PLACEMENT_3D('',#38478,#21638,#21639);
#17710=AXIS2_PLACEMENT_3D('',#38479,#21640,#21641);
#17711=AXIS2_PLACEMENT_3D('',#38480,#21642,#21643);
#17712=AXIS2_PLACEMENT_3D('',#38481,#21644,#21645);
#17713=AXIS2_PLACEMENT_3D('',#38482,#21646,#21647);
#17714=AXIS2_PLACEMENT_3D('',#38483,#21648,#21649);
#17715=AXIS2_PLACEMENT_3D('',#38484,#21650,#21651);
#17716=AXIS2_PLACEMENT_3D('',#38485,#21652,#21653);
#17717=AXIS2_PLACEMENT_3D('',#38486,#21654,#21655);
#17718=AXIS2_PLACEMENT_3D('',#38487,#21656,#21657);
#17719=AXIS2_PLACEMENT_3D('',#38488,#21658,#21659);
#17720=AXIS2_PLACEMENT_3D('',#38489,#21660,#21661);
#17721=AXIS2_PLACEMENT_3D('',#38490,#21662,#21663);
#17722=AXIS2_PLACEMENT_3D('',#38491,#21664,#21665);
#17723=AXIS2_PLACEMENT_3D('',#38492,#21666,#21667);
#17724=AXIS2_PLACEMENT_3D('',#38493,#21668,#21669);
#17725=AXIS2_PLACEMENT_3D('',#38494,#21670,#21671);
#17726=AXIS2_PLACEMENT_3D('',#38495,#21672,#21673);
#17727=AXIS2_PLACEMENT_3D('',#38496,#21674,#21675);
#17728=AXIS2_PLACEMENT_3D('',#38497,#21676,#21677);
#17729=AXIS2_PLACEMENT_3D('',#38498,#21678,#21679);
#17730=AXIS2_PLACEMENT_3D('',#38499,#21680,#21681);
#17731=AXIS2_PLACEMENT_3D('',#38500,#21682,#21683);
#17732=AXIS2_PLACEMENT_3D('',#38501,#21684,#21685);
#17733=AXIS2_PLACEMENT_3D('',#38502,#21686,#21687);
#17734=AXIS2_PLACEMENT_3D('',#38503,#21688,#21689);
#17735=AXIS2_PLACEMENT_3D('',#38504,#21690,#21691);
#17736=AXIS2_PLACEMENT_3D('',#38505,#21692,#21693);
#17737=AXIS2_PLACEMENT_3D('',#38506,#21694,#21695);
#17738=AXIS2_PLACEMENT_3D('',#38507,#21696,#21697);
#17739=AXIS2_PLACEMENT_3D('',#38508,#21698,#21699);
#17740=AXIS2_PLACEMENT_3D('',#38509,#21700,#21701);
#17741=AXIS2_PLACEMENT_3D('',#38510,#21702,#21703);
#17742=AXIS2_PLACEMENT_3D('',#38511,#21704,#21705);
#17743=AXIS2_PLACEMENT_3D('',#38512,#21706,#21707);
#17744=AXIS2_PLACEMENT_3D('',#38513,#21708,#21709);
#17745=AXIS2_PLACEMENT_3D('',#38514,#21710,#21711);
#17746=AXIS2_PLACEMENT_3D('',#38515,#21712,#21713);
#17747=AXIS2_PLACEMENT_3D('',#38516,#21714,#21715);
#17748=AXIS2_PLACEMENT_3D('',#38517,#21716,#21717);
#17749=AXIS2_PLACEMENT_3D('',#38518,#21718,#21719);
#17750=AXIS2_PLACEMENT_3D('',#38519,#21720,#21721);
#17751=AXIS2_PLACEMENT_3D('',#38520,#21722,#21723);
#17752=AXIS2_PLACEMENT_3D('',#38521,#21724,#21725);
#17753=AXIS2_PLACEMENT_3D('',#38522,#21726,#21727);
#17754=AXIS2_PLACEMENT_3D('',#38523,#21728,#21729);
#17755=AXIS2_PLACEMENT_3D('',#38524,#21730,#21731);
#17756=AXIS2_PLACEMENT_3D('',#38525,#21732,#21733);
#17757=AXIS2_PLACEMENT_3D('',#38526,#21734,#21735);
#17758=AXIS2_PLACEMENT_3D('',#38527,#21736,#21737);
#17759=AXIS2_PLACEMENT_3D('',#38528,#21738,#21739);
#17760=AXIS2_PLACEMENT_3D('',#38529,#21740,#21741);
#17761=AXIS2_PLACEMENT_3D('',#38530,#21742,#21743);
#17762=AXIS2_PLACEMENT_3D('',#38531,#21744,#21745);
#17763=AXIS2_PLACEMENT_3D('',#38532,#21746,#21747);
#17764=AXIS2_PLACEMENT_3D('',#38533,#21748,#21749);
#17765=AXIS2_PLACEMENT_3D('',#38534,#21750,#21751);
#17766=AXIS2_PLACEMENT_3D('',#38535,#21752,#21753);
#17767=AXIS2_PLACEMENT_3D('',#38536,#21754,#21755);
#17768=AXIS2_PLACEMENT_3D('',#38537,#21756,#21757);
#17769=AXIS2_PLACEMENT_3D('',#38538,#21758,#21759);
#17770=AXIS2_PLACEMENT_3D('',#38539,#21760,#21761);
#17771=AXIS2_PLACEMENT_3D('',#38540,#21762,#21763);
#17772=AXIS2_PLACEMENT_3D('',#38541,#21764,#21765);
#17773=AXIS2_PLACEMENT_3D('',#38542,#21766,#21767);
#17774=AXIS2_PLACEMENT_3D('',#38545,#21769,#21770);
#17775=AXIS2_PLACEMENT_3D('',#38546,#21771,#21772);
#17776=AXIS2_PLACEMENT_3D('',#38548,#21773,#21774);
#17777=AXIS2_PLACEMENT_3D('',#38549,#21775,#21776);
#17778=AXIS2_PLACEMENT_3D('',#38551,#21778,#21779);
#17779=AXIS2_PLACEMENT_3D('',#38552,#21780,#21781);
#17780=AXIS2_PLACEMENT_3D('',#38553,#21782,#21783);
#17781=AXIS2_PLACEMENT_3D('',#38554,#21784,#21785);
#17782=AXIS2_PLACEMENT_3D('',#38556,#21786,#21787);
#17783=AXIS2_PLACEMENT_3D('',#38558,#21789,#21790);
#21372=DIRECTION('axis',(0.,0.,1.));
#21373=DIRECTION('refdir',(1.,0.,0.));
#21374=DIRECTION('center_axis',(0.,0.,1.));
#21375=DIRECTION('ref_axis',(1.,0.,0.));
#21376=DIRECTION('',(0.,0.,-1.));
#21377=DIRECTION('center_axis',(0.,0.,1.));
#21378=DIRECTION('ref_axis',(1.,0.,0.));
#21379=DIRECTION('center_axis',(0.,0.,1.));
#21380=DIRECTION('ref_axis',(1.,0.,0.));
#21381=DIRECTION('',(0.,0.,-1.));
#21382=DIRECTION('center_axis',(0.,0.,1.));
#21383=DIRECTION('ref_axis',(1.,0.,0.));
#21384=DIRECTION('',(0.,0.,-1.));
#21385=DIRECTION('center_axis',(0.,0.,1.));
#21386=DIRECTION('ref_axis',(1.,0.,0.));
#21387=DIRECTION('',(0.,0.,-1.));
#21388=DIRECTION('center_axis',(0.,0.,1.));
#21389=DIRECTION('ref_axis',(1.,0.,0.));
#21390=DIRECTION('',(0.,0.,-1.));
#21391=DIRECTION('center_axis',(0.,0.,1.));
#21392=DIRECTION('ref_axis',(1.,0.,0.));
#21393=DIRECTION('',(0.,0.,-1.));
#21394=DIRECTION('center_axis',(0.,0.,1.));
#21395=DIRECTION('ref_axis',(1.,0.,0.));
#21396=DIRECTION('',(0.,0.,-1.));
#21397=DIRECTION('center_axis',(0.,0.,1.));
#21398=DIRECTION('ref_axis',(1.,0.,0.));
#21399=DIRECTION('',(0.,0.,-1.));
#21400=DIRECTION('center_axis',(0.,0.,1.));
#21401=DIRECTION('ref_axis',(1.,0.,0.));
#21402=DIRECTION('',(0.,0.,-1.));
#21403=DIRECTION('center_axis',(0.,0.,1.));
#21404=DIRECTION('ref_axis',(1.,0.,0.));
#21405=DIRECTION('',(0.,0.,-1.));
#21406=DIRECTION('center_axis',(0.,0.,1.));
#21407=DIRECTION('ref_axis',(1.,0.,0.));
#21408=DIRECTION('',(0.,0.,-1.));
#21409=DIRECTION('center_axis',(0.,0.,1.));
#21410=DIRECTION('ref_axis',(-0.266007747734115,-0.963970890714768,0.));
#21411=DIRECTION('',(0.,0.,1.));
#21412=DIRECTION('center_axis',(0.,0.,1.));
#21413=DIRECTION('ref_axis',(1.,5.3862180848358E-14,0.));
#21414=DIRECTION('center_axis',(0.,0.,1.));
#21415=DIRECTION('ref_axis',(1.,5.3862180848358E-14,0.));
#21416=DIRECTION('',(0.,0.,1.));
#21417=DIRECTION('center_axis',(0.,0.,1.));
#21418=DIRECTION('ref_axis',(1.,5.3862180848358E-14,0.));
#21419=DIRECTION('',(0.,0.,1.));
#21420=DIRECTION('center_axis',(0.,0.,1.));
#21421=DIRECTION('ref_axis',(1.,5.3862180848358E-14,0.));
#21422=DIRECTION('',(0.,0.,1.));
#21423=DIRECTION('center_axis',(0.,0.,1.));
#21424=DIRECTION('ref_axis',(1.,5.3862180848358E-14,0.));
#21425=DIRECTION('',(0.,0.,1.));
#21426=DIRECTION('center_axis',(0.,0.,1.));
#21427=DIRECTION('ref_axis',(1.,5.3862180848358E-14,0.));
#21428=DIRECTION('',(0.,0.,1.));
#21429=DIRECTION('center_axis',(0.,0.,1.));
#21430=DIRECTION('ref_axis',(1.,5.3862180848358E-14,0.));
#21431=DIRECTION('',(0.,0.,1.));
#21432=DIRECTION('center_axis',(0.,0.,1.));
#21433=DIRECTION('ref_axis',(1.,5.3862180848358E-14,0.));
#21434=DIRECTION('',(0.,0.,1.));
#21435=DIRECTION('center_axis',(0.,0.,1.));
#21436=DIRECTION('ref_axis',(1.,5.3862180848358E-14,0.));
#21437=DIRECTION('',(0.,0.,1.));
#21438=DIRECTION('center_axis',(0.,0.,1.));
#21439=DIRECTION('ref_axis',(1.,5.3862180848358E-14,0.));
#21440=DIRECTION('',(0.,0.,1.));
#21441=DIRECTION('center_axis',(0.,0.,1.));
#21442=DIRECTION('ref_axis',(1.,5.3862180848358E-14,0.));
#21443=DIRECTION('',(0.,0.,1.));
#21444=DIRECTION('center_axis',(0.,0.,1.));
#21445=DIRECTION('ref_axis',(1.,0.,0.));
#21446=DIRECTION('center_axis',(0.,0.,1.));
#21447=DIRECTION('ref_axis',(1.,0.,0.));
#21448=DIRECTION('center_axis',(0.,0.,1.));
#21449=DIRECTION('ref_axis',(1.,0.,0.));
#21450=DIRECTION('center_axis',(0.,0.,-1.));
#21451=DIRECTION('ref_axis',(1.,5.3862180848358E-14,0.));
#21452=DIRECTION('center_axis',(0.,0.,1.));
#21453=DIRECTION('ref_axis',(1.,5.3862180848358E-14,0.));
#21454=DIRECTION('center_axis',(0.0265854578674083,0.999646544249506,0.));
#21455=DIRECTION('ref_axis',(0.999646544249506,-0.0265854578674083,0.));
#21456=DIRECTION('',(0.,0.,-1.));
#21457=DIRECTION('',(0.,0.,-1.));
#21458=DIRECTION('center_axis',(-0.852426573191691,-0.522846954009173,0.));
#21459=DIRECTION('ref_axis',(-0.522846954009173,0.852426573191691,0.));
#21460=DIRECTION('',(0.,0.,1.));
#21461=DIRECTION('center_axis',(0.522846954009174,0.852426573191691,0.));
#21462=DIRECTION('ref_axis',(0.852426573191691,-0.522846954009174,0.));
#21463=DIRECTION('',(0.,0.,-1.));
#21464=DIRECTION('',(0.,0.,-1.));
#21465=DIRECTION('center_axis',(-0.999646544249506,-0.0265854578674079,
0.));
#21466=DIRECTION('ref_axis',(-0.0265854578674079,0.999646544249506,0.));
#21467=DIRECTION('',(0.,0.,1.));
#21468=DIRECTION('center_axis',(0.879012031059102,0.476799590240337,0.));
#21469=DIRECTION('ref_axis',(0.476799590240337,-0.879012031059102,0.));
#21470=DIRECTION('',(0.,0.,-1.));
#21471=DIRECTION('',(0.,0.,-1.));
#21472=DIRECTION('center_axis',(-0.879012031059104,0.476799590240333,0.));
#21473=DIRECTION('ref_axis',(0.476799590240333,0.879012031059104,0.));
#21474=DIRECTION('',(0.,0.,1.));
#21475=DIRECTION('center_axis',(0.999646544249506,-0.0265854578674083,0.));
#21476=DIRECTION('ref_axis',(-0.0265854578674083,-0.999646544249506,0.));
#21477=DIRECTION('',(0.,0.,-1.));
#21478=DIRECTION('',(0.,0.,-1.));
#21479=DIRECTION('center_axis',(-0.522846954009174,0.852426573191691,0.));
#21480=DIRECTION('ref_axis',(0.852426573191691,0.522846954009174,0.));
#21481=DIRECTION('',(0.,0.,1.));
#21482=DIRECTION('center_axis',(0.852426573191692,-0.522846954009172,0.));
#21483=DIRECTION('ref_axis',(-0.522846954009172,-0.852426573191692,0.));
#21484=DIRECTION('',(0.,0.,-1.));
#21485=DIRECTION('',(0.,0.,-1.));
#21486=DIRECTION('center_axis',(-0.026585457867411,0.999646544249506,0.));
#21487=DIRECTION('ref_axis',(0.999646544249506,0.026585457867411,0.));
#21488=DIRECTION('',(0.,0.,1.));
#21489=DIRECTION('center_axis',(0.476799590240335,-0.879012031059103,0.));
#21490=DIRECTION('ref_axis',(-0.879012031059103,-0.476799590240335,0.));
#21491=DIRECTION('',(0.,0.,-1.));
#21492=DIRECTION('',(0.,0.,-1.));
#21493=DIRECTION('center_axis',(0.476799590240335,0.879012031059103,0.));
#21494=DIRECTION('ref_axis',(0.879012031059103,-0.476799590240335,0.));
#21495=DIRECTION('',(0.,0.,1.));
#21496=DIRECTION('center_axis',(0.23304798366484,-0.972465237070073,0.));
#21497=DIRECTION('ref_axis',(-0.972465237070073,-0.23304798366484,0.));
#21498=DIRECTION('',(0.,0.,-1.));
#21499=DIRECTION('',(0.,0.,-1.));
#21500=DIRECTION('center_axis',(0.688058092689529,0.725655607767519,0.));
#21501=DIRECTION('ref_axis',(0.725655607767519,-0.688058092689529,0.));
#21502=DIRECTION('',(0.,0.,1.));
#21503=DIRECTION('center_axis',(-0.284407144380544,-0.958703591432359,0.));
#21504=DIRECTION('ref_axis',(-0.958703591432359,0.284407144380544,0.));
#21505=DIRECTION('',(0.,0.,-1.));
#21506=DIRECTION('',(0.,0.,-1.));
#21507=DIRECTION('center_axis',(0.95870359143236,0.284407144380544,0.));
#21508=DIRECTION('ref_axis',(0.284407144380544,-0.95870359143236,0.));
#21509=DIRECTION('',(0.,0.,1.));
#21510=DIRECTION('center_axis',(-0.725655607767519,-0.688058092689529,0.));
#21511=DIRECTION('ref_axis',(-0.688058092689529,0.725655607767519,0.));
#21512=DIRECTION('',(0.,0.,-1.));
#21513=DIRECTION('',(0.,0.,-1.));
#21514=DIRECTION('center_axis',(0.972465237070073,-0.23304798366484,0.));
#21515=DIRECTION('ref_axis',(-0.23304798366484,-0.972465237070073,0.));
#21516=DIRECTION('',(0.,0.,1.));
#21517=DIRECTION('center_axis',(-0.972465237070073,-0.23304798366484,0.));
#21518=DIRECTION('ref_axis',(-0.23304798366484,0.972465237070073,0.));
#21519=DIRECTION('',(0.,0.,-1.));
#21520=DIRECTION('',(0.,0.,-1.));
#21521=DIRECTION('center_axis',(0.725655607767519,-0.688058092689529,0.));
#21522=DIRECTION('ref_axis',(-0.688058092689529,-0.725655607767519,0.));
#21523=DIRECTION('',(0.,0.,1.));
#21524=DIRECTION('center_axis',(-0.95870359143236,0.284407144380544,0.));
#21525=DIRECTION('ref_axis',(0.284407144380544,0.95870359143236,0.));
#21526=DIRECTION('',(0.,0.,-1.));
#21527=DIRECTION('',(0.,0.,-1.));
#21528=DIRECTION('center_axis',(0.284407144380544,-0.95870359143236,0.));
#21529=DIRECTION('ref_axis',(-0.95870359143236,-0.284407144380544,0.));
#21530=DIRECTION('',(0.,0.,1.));
#21531=DIRECTION('center_axis',(-0.688058092689529,0.725655607767519,0.));
#21532=DIRECTION('ref_axis',(0.725655607767519,0.688058092689529,0.));
#21533=DIRECTION('',(0.,0.,-1.));
#21534=DIRECTION('',(0.,0.,-1.));
#21535=DIRECTION('center_axis',(-0.23304798366484,-0.972465237070073,0.));
#21536=DIRECTION('ref_axis',(-0.972465237070073,0.23304798366484,0.));
#21537=DIRECTION('',(0.,0.,1.));
#21538=DIRECTION('center_axis',(-0.852426573191692,0.522846954009171,0.));
#21539=DIRECTION('ref_axis',(0.522846954009171,0.852426573191692,0.));
#21540=DIRECTION('',(0.,0.,-1.));
#21541=DIRECTION('',(0.,0.,-1.));
#21542=DIRECTION('center_axis',(0.026585457867411,-0.999646544249506,0.));
#21543=DIRECTION('ref_axis',(-0.999646544249506,-0.026585457867411,0.));
#21544=DIRECTION('',(0.,0.,1.));
#21545=DIRECTION('center_axis',(-0.999646544249506,0.0265854578674102,0.));
#21546=DIRECTION('ref_axis',(0.0265854578674102,0.999646544249506,0.));
#21547=DIRECTION('',(0.,0.,-1.));
#21548=DIRECTION('',(0.,0.,-1.));
#21549=DIRECTION('center_axis',(0.522846954009173,-0.852426573191692,0.));
#21550=DIRECTION('ref_axis',(-0.852426573191692,-0.522846954009173,0.));
#21551=DIRECTION('',(0.,0.,1.));
#21552=DIRECTION('center_axis',(-0.879012031059103,-0.476799590240335,0.));
#21553=DIRECTION('ref_axis',(-0.476799590240335,0.879012031059103,0.));
#21554=DIRECTION('',(0.,0.,-1.));
#21555=DIRECTION('',(0.,0.,-1.));
#21556=DIRECTION('center_axis',(0.879012031059103,-0.476799590240335,0.));
#21557=DIRECTION('ref_axis',(-0.476799590240335,-0.879012031059103,0.));
#21558=DIRECTION('',(0.,0.,1.));
#21559=DIRECTION('center_axis',(-0.522846954009172,-0.852426573191692,0.));
#21560=DIRECTION('ref_axis',(-0.852426573191692,0.522846954009172,0.));
#21561=DIRECTION('',(0.,0.,-1.));
#21562=DIRECTION('',(0.,0.,-1.));
#21563=DIRECTION('center_axis',(0.999646544249506,0.0265854578674102,0.));
#21564=DIRECTION('ref_axis',(0.0265854578674102,-0.999646544249506,0.));
#21565=DIRECTION('',(0.,0.,1.));
#21566=DIRECTION('center_axis',(-0.0265854578674106,-0.999646544249506,
0.));
#21567=DIRECTION('ref_axis',(-0.999646544249506,0.0265854578674106,0.));
#21568=DIRECTION('',(0.,0.,-1.));
#21569=DIRECTION('',(0.,0.,-1.));
#21570=DIRECTION('center_axis',(0.852426573191692,0.522846954009171,0.));
#21571=DIRECTION('ref_axis',(0.522846954009171,-0.852426573191692,0.));
#21572=DIRECTION('',(0.,0.,1.));
#21573=DIRECTION('center_axis',(-0.476799590240335,0.879012031059103,0.));
#21574=DIRECTION('ref_axis',(0.879012031059103,0.476799590240335,0.));
#21575=DIRECTION('',(0.,0.,-1.));
#21576=DIRECTION('',(0.,0.,-1.));
#21577=DIRECTION('center_axis',(-0.476799590240335,-0.879012031059103,0.));
#21578=DIRECTION('ref_axis',(-0.879012031059103,0.476799590240335,0.));
#21579=DIRECTION('',(0.,0.,1.));
#21580=DIRECTION('center_axis',(0.688058092689529,-0.725655607767519,0.));
#21581=DIRECTION('ref_axis',(-0.725655607767519,-0.688058092689529,0.));
#21582=DIRECTION('',(0.,0.,-1.));
#21583=DIRECTION('',(0.,0.,-1.));
#21584=DIRECTION('center_axis',(0.23304798366484,0.972465237070073,0.));
#21585=DIRECTION('ref_axis',(0.972465237070073,-0.23304798366484,0.));
#21586=DIRECTION('',(0.,0.,1.));
#21587=DIRECTION('center_axis',(0.95870359143236,-0.284407144380542,0.));
#21588=DIRECTION('ref_axis',(-0.284407144380542,-0.95870359143236,0.));
#21589=DIRECTION('',(0.,0.,-1.));
#21590=DIRECTION('',(0.,0.,-1.));
#21591=DIRECTION('center_axis',(-0.284407144380544,0.95870359143236,0.));
#21592=DIRECTION('ref_axis',(0.95870359143236,0.284407144380544,0.));
#21593=DIRECTION('',(0.,0.,1.));
#21594=DIRECTION('center_axis',(0.972465237070073,0.233047983664838,0.));
#21595=DIRECTION('ref_axis',(0.233047983664838,-0.972465237070073,0.));
#21596=DIRECTION('',(0.,0.,-1.));
#21597=DIRECTION('',(0.,0.,-1.));
#21598=DIRECTION('center_axis',(-0.725655607767518,0.688058092689531,0.));
#21599=DIRECTION('ref_axis',(0.688058092689531,0.725655607767518,0.));
#21600=DIRECTION('',(0.,0.,1.));
#21601=DIRECTION('center_axis',(0.725655607767518,0.688058092689531,0.));
#21602=DIRECTION('ref_axis',(0.688058092689531,-0.725655607767518,0.));
#21603=DIRECTION('',(0.,0.,-1.));
#21604=DIRECTION('',(0.,0.,-1.));
#21605=DIRECTION('center_axis',(-0.972465237070073,0.233047983664838,0.));
#21606=DIRECTION('ref_axis',(0.233047983664838,0.972465237070073,0.));
#21607=DIRECTION('',(0.,0.,1.));
#21608=DIRECTION('center_axis',(0.284407144380542,0.95870359143236,0.));
#21609=DIRECTION('ref_axis',(0.95870359143236,-0.284407144380542,0.));
#21610=DIRECTION('',(0.,0.,-1.));
#21611=DIRECTION('',(0.,0.,-1.));
#21612=DIRECTION('center_axis',(-0.958703591432359,-0.284407144380547,0.));
#21613=DIRECTION('ref_axis',(-0.284407144380547,0.958703591432359,0.));
#21614=DIRECTION('',(0.,0.,1.));
#21615=DIRECTION('center_axis',(-0.233047983664838,0.972465237070073,0.));
#21616=DIRECTION('ref_axis',(0.972465237070073,0.233047983664838,0.));
#21617=DIRECTION('',(0.,0.,-1.));
#21618=DIRECTION('',(0.,0.,-1.));
#21619=DIRECTION('center_axis',(-0.688058092689531,-0.725655607767518,0.));
#21620=DIRECTION('ref_axis',(-0.725655607767518,0.688058092689531,0.));
#21621=DIRECTION('',(0.,0.,1.));
#21622=DIRECTION('center_axis',(0.,0.,1.));
#21623=DIRECTION('ref_axis',(1.,0.,0.));
#21624=DIRECTION('center_axis',(0.,0.,1.));
#21625=DIRECTION('ref_axis',(1.,0.,0.));
#21626=DIRECTION('center_axis',(0.,0.,1.));
#21627=DIRECTION('ref_axis',(1.,0.,0.));
#21628=DIRECTION('center_axis',(0.,0.,1.));
#21629=DIRECTION('ref_axis',(1.,0.,0.));
#21630=DIRECTION('center_axis',(0.,0.,1.));
#21631=DIRECTION('ref_axis',(1.,0.,0.));
#21632=DIRECTION('center_axis',(0.,0.,1.));
#21633=DIRECTION('ref_axis',(1.,0.,0.));
#21634=DIRECTION('center_axis',(0.,0.,1.));
#21635=DIRECTION('ref_axis',(1.,0.,0.));
#21636=DIRECTION('center_axis',(0.,0.,1.));
#21637=DIRECTION('ref_axis',(1.,0.,0.));
#21638=DIRECTION('center_axis',(0.,0.,1.));
#21639=DIRECTION('ref_axis',(1.,0.,0.));
#21640=DIRECTION('center_axis',(0.,0.,1.));
#21641=DIRECTION('ref_axis',(1.,0.,0.));
#21642=DIRECTION('center_axis',(0.,0.,1.));
#21643=DIRECTION('ref_axis',(1.,0.,0.));
#21644=DIRECTION('center_axis',(0.,0.,1.));
#21645=DIRECTION('ref_axis',(1.,0.,0.));
#21646=DIRECTION('center_axis',(0.,0.,1.));
#21647=DIRECTION('ref_axis',(1.,0.,0.));
#21648=DIRECTION('center_axis',(0.,0.,1.));
#21649=DIRECTION('ref_axis',(1.,0.,0.));
#21650=DIRECTION('center_axis',(0.,0.,1.));
#21651=DIRECTION('ref_axis',(1.,0.,0.));
#21652=DIRECTION('center_axis',(0.,0.,1.));
#21653=DIRECTION('ref_axis',(1.,0.,0.));
#21654=DIRECTION('center_axis',(0.,0.,1.));
#21655=DIRECTION('ref_axis',(1.,0.,0.));
#21656=DIRECTION('center_axis',(0.,0.,1.));
#21657=DIRECTION('ref_axis',(1.,0.,0.));
#21658=DIRECTION('center_axis',(0.,0.,1.));
#21659=DIRECTION('ref_axis',(1.,0.,0.));
#21660=DIRECTION('center_axis',(0.,0.,1.));
#21661=DIRECTION('ref_axis',(1.,0.,0.));
#21662=DIRECTION('center_axis',(0.,0.,1.));
#21663=DIRECTION('ref_axis',(1.,0.,0.));
#21664=DIRECTION('center_axis',(0.,0.,1.));
#21665=DIRECTION('ref_axis',(1.,0.,0.));
#21666=DIRECTION('center_axis',(0.,0.,1.));
#21667=DIRECTION('ref_axis',(1.,0.,0.));
#21668=DIRECTION('center_axis',(0.,0.,1.));
#21669=DIRECTION('ref_axis',(1.,0.,0.));
#21670=DIRECTION('center_axis',(0.,0.,1.));
#21671=DIRECTION('ref_axis',(1.,0.,0.));
#21672=DIRECTION('center_axis',(0.,0.,1.));
#21673=DIRECTION('ref_axis',(1.,0.,0.));
#21674=DIRECTION('center_axis',(0.,0.,1.));
#21675=DIRECTION('ref_axis',(1.,0.,0.));
#21676=DIRECTION('center_axis',(0.,0.,1.));
#21677=DIRECTION('ref_axis',(1.,0.,0.));
#21678=DIRECTION('center_axis',(0.,0.,1.));
#21679=DIRECTION('ref_axis',(1.,0.,0.));
#21680=DIRECTION('center_axis',(0.,0.,1.));
#21681=DIRECTION('ref_axis',(1.,0.,0.));
#21682=DIRECTION('center_axis',(0.,0.,1.));
#21683=DIRECTION('ref_axis',(1.,0.,0.));
#21684=DIRECTION('center_axis',(0.,0.,1.));
#21685=DIRECTION('ref_axis',(1.,0.,0.));
#21686=DIRECTION('center_axis',(0.,0.,1.));
#21687=DIRECTION('ref_axis',(1.,0.,0.));
#21688=DIRECTION('center_axis',(0.,0.,1.));
#21689=DIRECTION('ref_axis',(1.,0.,0.));
#21690=DIRECTION('center_axis',(0.,0.,1.));
#21691=DIRECTION('ref_axis',(1.,0.,0.));
#21692=DIRECTION('center_axis',(0.,0.,1.));
#21693=DIRECTION('ref_axis',(1.,0.,0.));
#21694=DIRECTION('center_axis',(0.,0.,1.));
#21695=DIRECTION('ref_axis',(1.,0.,0.));
#21696=DIRECTION('center_axis',(0.,0.,1.));
#21697=DIRECTION('ref_axis',(1.,0.,0.));
#21698=DIRECTION('center_axis',(0.,0.,1.));
#21699=DIRECTION('ref_axis',(1.,0.,0.));
#21700=DIRECTION('center_axis',(0.,0.,1.));
#21701=DIRECTION('ref_axis',(1.,0.,0.));
#21702=DIRECTION('center_axis',(0.,0.,1.));
#21703=DIRECTION('ref_axis',(1.,0.,0.));
#21704=DIRECTION('center_axis',(0.,0.,1.));
#21705=DIRECTION('ref_axis',(1.,0.,0.));
#21706=DIRECTION('center_axis',(0.,0.,1.));
#21707=DIRECTION('ref_axis',(1.,0.,0.));
#21708=DIRECTION('center_axis',(0.,0.,1.));
#21709=DIRECTION('ref_axis',(1.,0.,0.));
#21710=DIRECTION('center_axis',(0.,0.,1.));
#21711=DIRECTION('ref_axis',(1.,0.,0.));
#21712=DIRECTION('center_axis',(0.,0.,1.));
#21713=DIRECTION('ref_axis',(1.,0.,0.));
#21714=DIRECTION('center_axis',(0.,0.,1.));
#21715=DIRECTION('ref_axis',(1.,0.,0.));
#21716=DIRECTION('center_axis',(0.,0.,1.));
#21717=DIRECTION('ref_axis',(1.,0.,0.));
#21718=DIRECTION('center_axis',(0.,0.,1.));
#21719=DIRECTION('ref_axis',(1.,0.,0.));
#21720=DIRECTION('center_axis',(0.,0.,1.));
#21721=DIRECTION('ref_axis',(1.,0.,0.));
#21722=DIRECTION('center_axis',(0.,0.,1.));
#21723=DIRECTION('ref_axis',(1.,0.,0.));
#21724=DIRECTION('center_axis',(0.,0.,1.));
#21725=DIRECTION('ref_axis',(1.,0.,0.));
#21726=DIRECTION('center_axis',(0.,0.,1.));
#21727=DIRECTION('ref_axis',(1.,0.,0.));
#21728=DIRECTION('center_axis',(0.,0.,1.));
#21729=DIRECTION('ref_axis',(1.,0.,0.));
#21730=DIRECTION('center_axis',(0.,0.,1.));
#21731=DIRECTION('ref_axis',(1.,0.,0.));
#21732=DIRECTION('center_axis',(0.,0.,1.));
#21733=DIRECTION('ref_axis',(1.,0.,0.));
#21734=DIRECTION('center_axis',(0.,0.,1.));
#21735=DIRECTION('ref_axis',(1.,0.,0.));
#21736=DIRECTION('center_axis',(0.,0.,1.));
#21737=DIRECTION('ref_axis',(1.,0.,0.));
#21738=DIRECTION('center_axis',(0.,0.,1.));
#21739=DIRECTION('ref_axis',(1.,0.,0.));
#21740=DIRECTION('center_axis',(0.,0.,1.));
#21741=DIRECTION('ref_axis',(1.,0.,0.));
#21742=DIRECTION('center_axis',(0.,0.,1.));
#21743=DIRECTION('ref_axis',(1.,0.,0.));
#21744=DIRECTION('center_axis',(0.,0.,1.));
#21745=DIRECTION('ref_axis',(1.,0.,0.));
#21746=DIRECTION('center_axis',(0.,0.,1.));
#21747=DIRECTION('ref_axis',(1.,0.,0.));
#21748=DIRECTION('center_axis',(0.,0.,1.));
#21749=DIRECTION('ref_axis',(1.,0.,0.));
#21750=DIRECTION('center_axis',(0.,0.,1.));
#21751=DIRECTION('ref_axis',(1.,0.,0.));
#21752=DIRECTION('center_axis',(0.,0.,1.));
#21753=DIRECTION('ref_axis',(1.,0.,0.));
#21754=DIRECTION('center_axis',(0.,0.,1.));
#21755=DIRECTION('ref_axis',(1.,0.,0.));
#21756=DIRECTION('center_axis',(0.,0.,1.));
#21757=DIRECTION('ref_axis',(1.,0.,0.));
#21758=DIRECTION('center_axis',(0.,0.,1.));
#21759=DIRECTION('ref_axis',(1.,0.,0.));
#21760=DIRECTION('center_axis',(0.,0.,1.));
#21761=DIRECTION('ref_axis',(1.,0.,0.));
#21762=DIRECTION('center_axis',(0.,0.,1.));
#21763=DIRECTION('ref_axis',(1.,0.,0.));
#21764=DIRECTION('center_axis',(0.,0.,1.));
#21765=DIRECTION('ref_axis',(1.,0.,0.));
#21766=DIRECTION('center_axis',(0.,0.,1.));
#21767=DIRECTION('ref_axis',(1.,0.,0.));
#21768=DIRECTION('',(0.707106781186548,8.65956056235494E-17,-0.707106781186547));
#21769=DIRECTION('center_axis',(0.,0.,1.));
#21770=DIRECTION('ref_axis',(1.,0.,0.));
#21771=DIRECTION('center_axis',(0.,0.,-1.));
#21772=DIRECTION('ref_axis',(-1.,0.,0.));
#21773=DIRECTION('center_axis',(0.,0.,1.));
#21774=DIRECTION('ref_axis',(1.,0.,0.));
#21775=DIRECTION('center_axis',(0.,0.,1.));
#21776=DIRECTION('ref_axis',(1.,0.,0.));
#21777=DIRECTION('',(0.707106781186547,8.65956056235493E-17,-0.707106781186547));
#21778=DIRECTION('center_axis',(0.,0.,1.));
#21779=DIRECTION('ref_axis',(0.939073945770631,-0.343715179145143,0.));
#21780=DIRECTION('center_axis',(0.,0.,1.));
#21781=DIRECTION('ref_axis',(1.,0.,0.));
#21782=DIRECTION('center_axis',(0.,0.,-1.));
#21783=DIRECTION('ref_axis',(-1.,0.,0.));
#21784=DIRECTION('center_axis',(0.,0.,-1.));
#21785=DIRECTION('ref_axis',(1.,0.,0.));
#21786=DIRECTION('center_axis',(0.,0.,1.));
#21787=DIRECTION('ref_axis',(1.,0.,0.));
#21788=DIRECTION('',(-0.707106781186548,-8.65956056235494E-17,-0.707106781186547));
#21789=DIRECTION('center_axis',(0.,0.,1.));
#21790=DIRECTION('ref_axis',(1.,0.,0.));
#36255=CARTESIAN_POINT('',(0.,0.,0.));
#36256=CARTESIAN_POINT('Origin',(0.,0.,-0.385));
#36257=CARTESIAN_POINT('',(-0.195612035850383,0.000135947154934524,-0.752013030787577));
#36258=CARTESIAN_POINT('',(-0.195578202233822,0.00020702102411161,-0.762186969212424));
#36259=CARTESIAN_POINT('',(-0.1954,-2.39295984553393E-17,-0.385));
#36260=CARTESIAN_POINT('',(0.0862546024668518,0.17550570910154,-0.7746));
#36261=CARTESIAN_POINT('Ctrl Pts',(-0.195612035850383,0.000135947154934524,
-0.752013030787577));
#36262=CARTESIAN_POINT('Ctrl Pts',(-0.195667083286635,0.00761212544448936,
-0.752440649041024));
#36263=CARTESIAN_POINT('Ctrl Pts',(-0.19527544420465,0.0150821391217423,
-0.752868267294471));
#36264=CARTESIAN_POINT('Ctrl Pts',(-0.194417810721063,0.0224978227107708,
-0.753295885547918));
#36265=CARTESIAN_POINT('Ctrl Pts',(-0.187011858244344,0.0865347350909431,
-0.756988512437858));
#36266=CARTESIAN_POINT('Ctrl Pts',(-0.144857163949201,0.146520306506109,
-0.760681139327799));
#36267=CARTESIAN_POINT('Ctrl Pts',(-0.0871192266947845,0.175237646686046,
-0.76437376621774));
#36268=CARTESIAN_POINT('Ctrl Pts',(-0.0338200748021689,0.201747251098443,
-0.767782510811827));
#36269=CARTESIAN_POINT('Ctrl Pts',(0.0327583993499999,0.201611508316804,
-0.771191255405914));
#36270=CARTESIAN_POINT('Ctrl Pts',(0.0863566189666486,0.175629287040327,
-0.7746));
#36271=CARTESIAN_POINT('',(-0.0861525859670513,0.175382131162755,-0.7746));
#36272=CARTESIAN_POINT('Origin',(0.,0.,-0.7746));
#36273=CARTESIAN_POINT('Ctrl Pts',(-0.0861525859670512,0.175382131162755,
-0.7746));
#36274=CARTESIAN_POINT('Ctrl Pts',(-0.144282890666664,0.146826906980442,
-0.770907373110059));
#36275=CARTESIAN_POINT('Ctrl Pts',(-0.186613134667349,0.0873604776073136,
-0.767214746220119));
#36276=CARTESIAN_POINT('Ctrl Pts',(-0.194290909418724,0.023452807632156,
-0.763522119330178));
#36277=CARTESIAN_POINT('Ctrl Pts',(-0.195216265284969,0.0157504017626666,
-0.763077069290927));
#36278=CARTESIAN_POINT('Ctrl Pts',(-0.195638258465322,0.00798348231459053,
-0.762632019251675));
#36279=CARTESIAN_POINT('Ctrl Pts',(-0.195578202233822,0.00020702102411161,
-0.762186969212424));
#36280=CARTESIAN_POINT('Origin',(0.,0.,-0.385));
#36281=CARTESIAN_POINT('',(-0.195106158228715,6.7253471116302E-5,-0.682013030787577));
#36282=CARTESIAN_POINT('',(-0.195102641109175,6.37944958194417E-5,-0.692186969212424));
#36283=CARTESIAN_POINT('',(-0.1954,-2.39295984553393E-17,-0.385));
#36284=CARTESIAN_POINT('Ctrl Pts',(-0.195106158228715,6.7253471116302E-5,
-0.682013030787577));
#36285=CARTESIAN_POINT('Ctrl Pts',(-0.195193741697796,0.0283198531480969,
-0.683618221034713));
#36286=CARTESIAN_POINT('Ctrl Pts',(-0.18945610577258,0.0565385117234044,
-0.685223411281848));
#36287=CARTESIAN_POINT('Ctrl Pts',(-0.177715395582584,0.0819875737941825,
-0.686828601528984));
#36288=CARTESIAN_POINT('Ctrl Pts',(-0.150706720298178,0.140531345221913,
-0.690521228418925));
#36289=CARTESIAN_POINT('Ctrl Pts',(-0.0919299226246749,0.184418479592776,
-0.694213855308865));
#36290=CARTESIAN_POINT('Ctrl Pts',(-0.0281252717103119,0.19368402419514,
-0.697906482198806));
#36291=CARTESIAN_POINT('Ctrl Pts',(0.0356793792040508,0.202949568797503,
-0.701599109088747));
#36292=CARTESIAN_POINT('Ctrl Pts',(0.104511883359273,0.177593523631367,
-0.705291735978687));
#36293=CARTESIAN_POINT('Ctrl Pts',(0.147056344142496,0.129148732777355,
-0.708984362868628));
#36294=CARTESIAN_POINT('Ctrl Pts',(0.189600804925718,0.080703941923342,
-0.712676989758569));
#36295=CARTESIAN_POINT('Ctrl Pts',(0.20585722233694,0.00917040538145272,
-0.71636961664851));
#36296=CARTESIAN_POINT('Ctrl Pts',(0.1884307024384,-0.0529021236960677,
-0.720062243538451));
#36297=CARTESIAN_POINT('Ctrl Pts',(0.171004182539859,-0.114974652773588,
-0.723754870428392));
#36298=CARTESIAN_POINT('Ctrl Pts',(0.119894725331557,-0.16758617438674,
-0.727447497318332));
#36299=CARTESIAN_POINT('Ctrl Pts',(0.0583527546211337,-0.186811585253294,
-0.731140124208273));
#36300=CARTESIAN_POINT('Ctrl Pts',(-0.00318921608928925,-0.206036996119848,
-0.734832751098214));
#36301=CARTESIAN_POINT('Ctrl Pts',(-0.0751637003018327,-0.191876296239803,
-0.738525377988155));
#36302=CARTESIAN_POINT('Ctrl Pts',(-0.124822337078956,-0.150751819627192,
-0.742218004878095));
#36303=CARTESIAN_POINT('Ctrl Pts',(-0.168730341539278,-0.114389691712985,
-0.745483013514589));
#36304=CARTESIAN_POINT('Ctrl Pts',(-0.195191730231224,-0.0569471789431846,
-0.748748022151083));
#36305=CARTESIAN_POINT('Ctrl Pts',(-0.195612035850383,0.000135947154934524,
-0.752013030787577));
#36306=CARTESIAN_POINT('Ctrl Pts',(-0.195578202233822,0.00020702102411161,
-0.762186969212424));
#36307=CARTESIAN_POINT('Ctrl Pts',(-0.195139965608823,-0.056538633261677,
-0.758939392361734));
#36308=CARTESIAN_POINT('Ctrl Pts',(-0.1690336868213,-0.113792369099031,
-0.755691815511045));
#36309=CARTESIAN_POINT('Ctrl Pts',(-0.125540731300798,-0.150194679039488,
-0.752444238660355));
#36310=CARTESIAN_POINT('Ctrl Pts',(-0.0760874729294314,-0.191585585158787,
-0.748751611770415));
#36311=CARTESIAN_POINT('Ctrl Pts',(-0.00415565068463411,-0.206018486820197,
-0.745058984880474));
#36312=CARTESIAN_POINT('Ctrl Pts',(0.0574817652959297,-0.187066360843203,
-0.741366357990533));
#36313=CARTESIAN_POINT('Ctrl Pts',(0.119119181276493,-0.168114234866209,
-0.737673731100593));
#36314=CARTESIAN_POINT('Ctrl Pts',(0.170462190992824,-0.11577708125081,
-0.733981104210652));
#36315=CARTESIAN_POINT('Ctrl Pts',(0.188176832473196,-0.0537951148800162,
-0.730288477320711));
#36316=CARTESIAN_POINT('Ctrl Pts',(0.205891473953568,0.00818685149077737,
-0.72659585043077));
#36317=CARTESIAN_POINT('Ctrl Pts',(0.189977747197981,0.0798136306169658,
-0.722903223540829));
#36318=CARTESIAN_POINT('Ctrl Pts',(0.147662757203391,0.128461801942711,
-0.719210596650889));
#36319=CARTESIAN_POINT('Ctrl Pts',(0.1053477672088,0.177109973268457,-0.715517969760948));
#36320=CARTESIAN_POINT('Ctrl Pts',(0.036631513975206,0.202779536793759,
-0.711825342871007));
#36321=CARTESIAN_POINT('Ctrl Pts',(-0.0272167615306242,0.193811384880893,
-0.708132715981067));
#36322=CARTESIAN_POINT('Ctrl Pts',(-0.0910650370364544,0.184843232968026,
-0.704440089091126));
#36323=CARTESIAN_POINT('Ctrl Pts',(-0.150045334814521,0.14123736561699,
-0.700747462201185));
#36324=CARTESIAN_POINT('Ctrl Pts',(-0.177328074880872,0.0828221813027525,
-0.697054835311244));
#36325=CARTESIAN_POINT('Ctrl Pts',(-0.189316715073911,0.0571532556431493,
-0.695432213278304));
#36326=CARTESIAN_POINT('Ctrl Pts',(-0.195184816078502,0.028624771980631,
-0.693809591245364));
#36327=CARTESIAN_POINT('Ctrl Pts',(-0.195102641109175,6.37944958194417E-5,
-0.692186969212424));
#36328=CARTESIAN_POINT('Origin',(0.,0.,-0.385));
#36329=CARTESIAN_POINT('',(-0.195373814288334,-0.000175590164213202,-0.612013030787577));
#36330=CARTESIAN_POINT('',(-0.195382883542994,-0.000175680656981076,-0.622186969212423));
#36331=CARTESIAN_POINT('',(-0.1954,-2.39295984553393E-17,-0.385));
#36332=CARTESIAN_POINT('Ctrl Pts',(-0.195373814288334,-0.000175590164213202,
-0.612013030787577));
#36333=CARTESIAN_POINT('Ctrl Pts',(-0.194935462027994,0.0486337685077184,
-0.614795793028401));
#36334=CARTESIAN_POINT('Ctrl Pts',(-0.176386685151872,0.0977403470970804,
-0.617578555269226));
#36335=CARTESIAN_POINT('Ctrl Pts',(-0.143291075940014,0.133313048722114,
-0.62036131751005));
#36336=CARTESIAN_POINT('Ctrl Pts',(-0.0993743752166056,0.180516763305194,
-0.624053944399991));
#36337=CARTESIAN_POINT('Ctrl Pts',(-0.0298431035570151,0.203889554183137,
-0.627746571289932));
#36338=CARTESIAN_POINT('Ctrl Pts',(0.0336694536774745,0.192797988921239,
-0.631439198179872));
#36339=CARTESIAN_POINT('Ctrl Pts',(0.0971820109119643,0.181706423659341,
-0.635131825069813));
#36340=CARTESIAN_POINT('Ctrl Pts',(0.154675853721353,0.136150502257601,
-0.638824451959754));
#36341=CARTESIAN_POINT('Ctrl Pts',(0.179994115466673,0.0768558559611854,
-0.642517078849694));
#36342=CARTESIAN_POINT('Ctrl Pts',(0.205312377211992,0.0175612096647699,
-0.646209705739635));
#36343=CARTESIAN_POINT('Ctrl Pts',(0.198455057893242,-0.0554721615263214,
-0.649902332629576));
#36344=CARTESIAN_POINT('Ctrl Pts',(0.162541919102326,-0.109017568867995,
-0.653594959519517));
#36345=CARTESIAN_POINT('Ctrl Pts',(0.12662878031141,-0.162562976209668,
-0.657287586409458));
#36346=CARTESIAN_POINT('Ctrl Pts',(0.0616598220483278,-0.196620419701923,
-0.660980213299398));
#36347=CARTESIAN_POINT('Ctrl Pts',(-0.00280733049035602,-0.195695666682811,
-0.664672840189339));
#36348=CARTESIAN_POINT('Ctrl Pts',(-0.0672744830290399,-0.194770913663699,
-0.66836546707928));
#36349=CARTESIAN_POINT('Ctrl Pts',(-0.131239829843325,-0.15886396413322,
-0.67205809396922));
#36350=CARTESIAN_POINT('Ctrl Pts',(-0.165602226802813,-0.104310285125682,
-0.675750720859161));
#36351=CARTESIAN_POINT('Ctrl Pts',(-0.185027240129573,-0.073471169245769,
-0.677838157501967));
#36352=CARTESIAN_POINT('Ctrl Pts',(-0.194992262107684,-0.0366732587052289,
-0.679925594144772));
#36353=CARTESIAN_POINT('Ctrl Pts',(-0.195106158228715,6.7253471116302E-5,
-0.682013030787577));
#36354=CARTESIAN_POINT('Ctrl Pts',(-0.195102641109175,6.37944958194417E-5,
-0.692186969212424));
#36355=CARTESIAN_POINT('Ctrl Pts',(-0.194997809187644,-0.0363719008873622,
-0.690116964355423));
#36356=CARTESIAN_POINT('Ctrl Pts',(-0.185209193124591,-0.0728604783826336,
-0.688046959498422));
#36357=CARTESIAN_POINT('Ctrl Pts',(-0.166090287545791,-0.103532484641873,
-0.685976954641422));
#36358=CARTESIAN_POINT('Ctrl Pts',(-0.131984577789722,-0.158247464994821,
-0.682284327751481));
#36359=CARTESIAN_POINT('Ctrl Pts',(-0.0681879759229486,-0.194452924423278,
-0.67859170086154));
#36360=CARTESIAN_POINT('Ctrl Pts',(-0.00372575719310086,-0.195679956595876,
-0.674899073971599));
#36361=CARTESIAN_POINT('Ctrl Pts',(0.060736461536747,-0.196906988768474,
-0.671206447081658));
#36362=CARTESIAN_POINT('Ctrl Pts',(0.125864297129669,-0.163155593685212,
-0.667513820191718));
#36363=CARTESIAN_POINT('Ctrl Pts',(0.162028316469382,-0.109779523904799,
-0.663821193301777));
#36364=CARTESIAN_POINT('Ctrl Pts',(0.198192335809096,-0.0564034541243863,
-0.660128566411836));
#36365=CARTESIAN_POINT('Ctrl Pts',(0.205392538895601,0.0165972903531772,
-0.656435939521895));
#36366=CARTESIAN_POINT('Ctrl Pts',(0.180352920431713,0.0760102116200135,
-0.652743312631955));
#36367=CARTESIAN_POINT('Ctrl Pts',(0.155313301967824,0.13542313288685,-0.649050685742014));
#36368=CARTESIAN_POINT('Ctrl Pts',(0.0980338619535436,0.181248230942959,
-0.645358058852073));
#36369=CARTESIAN_POINT('Ctrl Pts',(0.0345740548428563,0.19263775515523,
-0.641665431962132));
#36370=CARTESIAN_POINT('Ctrl Pts',(-0.028885752267831,0.2040272793675,-0.637972805072192));
#36371=CARTESIAN_POINT('Ctrl Pts',(-0.0985259264749248,0.180981229735933,
-0.634280178182251));
#36372=CARTESIAN_POINT('Ctrl Pts',(-0.142663705648477,0.133984207668471,
-0.63058755129231));
#36373=CARTESIAN_POINT('Ctrl Pts',(-0.176134280736128,0.0983454105776664,
-0.627787357265681));
#36374=CARTESIAN_POINT('Ctrl Pts',(-0.194939710785028,0.0489336135733413,
-0.624987163239052));
#36375=CARTESIAN_POINT('Ctrl Pts',(-0.195382883542994,-0.000175680656981076,
-0.622186969212423));
#36376=CARTESIAN_POINT('Origin',(0.,0.,-0.385));
#36377=CARTESIAN_POINT('',(-0.195672562949621,8.22112365601695E-5,-0.542013030787577));
#36378=CARTESIAN_POINT('',(-0.195667167474188,8.703216064893E-5,-0.552186969212423));
#36379=CARTESIAN_POINT('',(-0.1954,-2.39295984553393E-17,-0.385));
#36380=CARTESIAN_POINT('Ctrl Pts',(-0.195672562949621,8.22112365601695E-5,
-0.542013030787577));
#36381=CARTESIAN_POINT('Ctrl Pts',(-0.195697468556697,0.00475918250908728,
-0.542280738132149));
#36382=CARTESIAN_POINT('Ctrl Pts',(-0.195544212090925,0.00943449414701473,
-0.542548445476721));
#36383=CARTESIAN_POINT('Ctrl Pts',(-0.195207549301115,0.0140965614284866,
-0.542816152821294));
#36384=CARTESIAN_POINT('Ctrl Pts',(-0.190563784026466,0.0784028845657411,
-0.546508779711234));
#36385=CARTESIAN_POINT('Ctrl Pts',(-0.151024907292751,0.140189320250109,
-0.550201406601176));
#36386=CARTESIAN_POINT('Ctrl Pts',(-0.0945791532634838,0.171346094632147,
-0.553894033491116));
#36387=CARTESIAN_POINT('Ctrl Pts',(-0.0381333992342172,0.202502869014184,
-0.557586660381057));
#36388=CARTESIAN_POINT('Ctrl Pts',(0.0352192320906011,0.20302998209389,
-0.561279287270997));
#36389=CARTESIAN_POINT('Ctrl Pts',(0.0921069201474241,0.172687624146735,
-0.564971914160938));
#36390=CARTESIAN_POINT('Ctrl Pts',(0.148994608204248,0.142345266199579,
-0.568664541050879));
#36391=CARTESIAN_POINT('Ctrl Pts',(0.189417352993076,0.0811334372255617,
-0.57235716794082));
#36392=CARTESIAN_POINT('Ctrl Pts',(0.194984803922326,0.0169004918108476,
-0.576049794830761));
#36393=CARTESIAN_POINT('Ctrl Pts',(0.200552254851577,-0.0473324536038658,
-0.579742421720702));
#36394=CARTESIAN_POINT('Ctrl Pts',(0.171264411921251,-0.114586515459276,
-0.583435048610642));
#36395=CARTESIAN_POINT('Ctrl Pts',(0.120445796091562,-0.154264418250576,
-0.587127675500583));
#36396=CARTESIAN_POINT('Ctrl Pts',(0.0696271802618727,-0.193942321041876,
-0.590820302390524));
#36397=CARTESIAN_POINT('Ctrl Pts',(-0.00272220846717902,-0.206044064769067,
-0.594512929280465));
#36398=CARTESIAN_POINT('Ctrl Pts',(-0.0636869760053119,-0.185063958956186,
-0.598205556170405));
#36399=CARTESIAN_POINT('Ctrl Pts',(-0.124651743543445,-0.164083853143304,
-0.601898183060346));
#36400=CARTESIAN_POINT('Ctrl Pts',(-0.174231889890659,-0.110021897790351,
-0.605590809950287));
#36401=CARTESIAN_POINT('Ctrl Pts',(-0.189870898170653,-0.0474736009697657,
-0.609283436840228));
#36402=CARTESIAN_POINT('Ctrl Pts',(-0.193724355669966,-0.0320616771995824,
-0.610193301489344));
#36403=CARTESIAN_POINT('Ctrl Pts',(-0.195517139945011,-0.0161345209525238,
-0.611103166138461));
#36404=CARTESIAN_POINT('Ctrl Pts',(-0.195373814288334,-0.000175590164213202,
-0.612013030787577));
#36405=CARTESIAN_POINT('Ctrl Pts',(-0.195382883542994,-0.000175680656981076,
-0.622186969212423));
#36406=CARTESIAN_POINT('Ctrl Pts',(-0.19552412444615,-0.0158270061181529,
-0.621294536349111));
#36407=CARTESIAN_POINT('Ctrl Pts',(-0.193800270478103,-0.0314476057070434,
-0.620402103485799));
#36408=CARTESIAN_POINT('Ctrl Pts',(-0.190091640716924,-0.0465818348493538,
-0.619509670622488));
#36409=CARTESIAN_POINT('Ctrl Pts',(-0.174746412471808,-0.109202860796361,
-0.615817043732547));
#36410=CARTESIAN_POINT('Ctrl Pts',(-0.125420571841566,-0.163496918187019,
-0.612124416842606));
#36411=CARTESIAN_POINT('Ctrl Pts',(-0.0645549580566868,-0.184762953588956,
-0.608431789952666));
#36412=CARTESIAN_POINT('Ctrl Pts',(-0.0036893442718077,-0.206028988990894,
-0.604739163062725));
#36413=CARTESIAN_POINT('Ctrl Pts',(0.0687160426677074,-0.19426700240411,
-0.601046536172783));
#36414=CARTESIAN_POINT('Ctrl Pts',(0.119720342167793,-0.154828085566673,
-0.597353909282843));
#36415=CARTESIAN_POINT('Ctrl Pts',(0.170724641667879,-0.115389168729235,
-0.593661282392902));
#36416=CARTESIAN_POINT('Ctrl Pts',(0.200327853728537,-0.0482733216411438,
-0.589968655502962));
#36417=CARTESIAN_POINT('Ctrl Pts',(0.195061974822576,0.015985047408839,
-0.586276028613022));
#36418=CARTESIAN_POINT('Ctrl Pts',(0.189796095916616,0.0802434164588218,
-0.582583401723081));
#36419=CARTESIAN_POINT('Ctrl Pts',(0.149661126044039,0.141644307470696,
-0.578890774833139));
#36420=CARTESIAN_POINT('Ctrl Pts',(0.092916495169642,0.172253359155183,
-0.575198147943198));
#36421=CARTESIAN_POINT('Ctrl Pts',(0.0361718642952446,0.20286241083967,
-0.571505521053257));
#36422=CARTESIAN_POINT('Ctrl Pts',(-0.0371824275809728,0.202679623196771,
-0.567812894163317));
#36423=CARTESIAN_POINT('Ctrl Pts',(-0.0937738058612257,0.171788151132837,
-0.564120267273376));
#36424=CARTESIAN_POINT('Ctrl Pts',(-0.150365184141479,0.140896679068903,
-0.560427640383436));
#36425=CARTESIAN_POINT('Ctrl Pts',(-0.190193648825767,0.0792965225839352,
-0.556735013493495));
#36426=CARTESIAN_POINT('Ctrl Pts',(-0.195139216797218,0.0150127096795879,
-0.553042386603554));
#36427=CARTESIAN_POINT('Ctrl Pts',(-0.195521106165581,0.010048809709412,
-0.552757247473177));
#36428=CARTESIAN_POINT('Ctrl Pts',(-0.195694999368898,0.00506890790750389,
-0.5524721083428));
#36429=CARTESIAN_POINT('Ctrl Pts',(-0.195667167474188,8.703216064893E-5,
-0.552186969212423));
#36430=CARTESIAN_POINT('Origin',(0.,0.,-0.385));
#36431=CARTESIAN_POINT('',(-0.195144246227183,0.000106621721020397,-0.472013030787577));
#36432=CARTESIAN_POINT('',(-0.195139240617864,0.000102604098994689,-0.482186969212423));
#36433=CARTESIAN_POINT('',(-0.1954,-2.39295984553393E-17,-0.385));
#36434=CARTESIAN_POINT('Ctrl Pts',(-0.195144246227183,0.000106621721020397,
-0.472013030787577));
#36435=CARTESIAN_POINT('Ctrl Pts',(-0.195271140890506,0.0255321757748805,
-0.473458310125838));
#36436=CARTESIAN_POINT('Ctrl Pts',(-0.190654961237712,0.0509134566429959,
-0.474903589464099));
#36437=CARTESIAN_POINT('Ctrl Pts',(-0.181080042024378,0.0742611522024674,
-0.476348868802359));
#36438=CARTESIAN_POINT('Ctrl Pts',(-0.156616532984865,0.133913515699754,
-0.4800414956923));
#36439=CARTESIAN_POINT('Ctrl Pts',(-0.0997833319551522,0.180291027942414,
-0.483734122582241));
#36440=CARTESIAN_POINT('Ctrl Pts',(-0.0364367355576039,0.19229421376834,
-0.487426749472182));
#36441=CARTESIAN_POINT('Ctrl Pts',(0.0269098608399439,0.204297399594266,
-0.491119376362123));
#36442=CARTESIAN_POINT('Ctrl Pts',(0.0967698526053274,0.181926259003459,
-0.494812003252064));
#36443=CARTESIAN_POINT('Ctrl Pts',(0.141360397382926,0.135358554943971,
-0.498504630142004));
#36444=CARTESIAN_POINT('Ctrl Pts',(0.185950942160524,0.0887908508844819,
-0.502197257031945));
#36445=CARTESIAN_POINT('Ctrl Pts',(0.205272039950337,0.0180265833563106,
-0.505889883921886));
#36446=CARTESIAN_POINT('Ctrl Pts',(0.190533546493163,-0.0447400045445576,
-0.509582510811826));
#36447=CARTESIAN_POINT('Ctrl Pts',(0.175795053035988,-0.107506592445426,
-0.513275137701767));
#36448=CARTESIAN_POINT('Ctrl Pts',(0.126996968331827,-0.162275500718991,
-0.516967764591708));
#36449=CARTESIAN_POINT('Ctrl Pts',(0.0663400083406457,-0.184129583838522,
-0.520660391481649));
#36450=CARTESIAN_POINT('Ctrl Pts',(0.00568304834946542,-0.205983666958053,
-0.52435301837159));
#36451=CARTESIAN_POINT('Ctrl Pts',(-0.0668327869287337,-0.19492292492355,
-0.528045645261531));
#36452=CARTESIAN_POINT('Ctrl Pts',(-0.118216377660041,-0.155979448611229,
-0.531738272151471));
#36453=CARTESIAN_POINT('Ctrl Pts',(-0.165874770845197,-0.119859288854497,
-0.53516319169684));
#36454=CARTESIAN_POINT('Ctrl Pts',(-0.195353932541471,-0.0597527191423684,
-0.538588111242208));
#36455=CARTESIAN_POINT('Ctrl Pts',(-0.195672562949621,8.22112365601695E-5,
-0.542013030787577));
#36456=CARTESIAN_POINT('Ctrl Pts',(-0.195667167474188,8.703216064893E-5,
-0.552186969212423));
#36457=CARTESIAN_POINT('Ctrl Pts',(-0.19533456899701,-0.059447696042551,
-0.548779481452859));
#36458=CARTESIAN_POINT('Ctrl Pts',(-0.166193851506661,-0.119264320953253,
-0.545371993693295));
#36459=CARTESIAN_POINT('Ctrl Pts',(-0.118947235469162,-0.155422811859585,
-0.541964505933731));
#36460=CARTESIAN_POINT('Ctrl Pts',(-0.0677470149110404,-0.194607051170686,
-0.538271879043791));
#36461=CARTESIAN_POINT('Ctrl Pts',(0.00471609746381744,-0.20600806046916,
-0.53457925215385));
#36462=CARTESIAN_POINT('Ctrl Pts',(0.0654749683434781,-0.184438943551293,
-0.530886625263909));
#36463=CARTESIAN_POINT('Ctrl Pts',(0.126233839223138,-0.162869826633425,
-0.527193998373969));
#36464=CARTESIAN_POINT('Ctrl Pts',(0.175288468607602,-0.108330583499217,
-0.523501371484028));
#36465=CARTESIAN_POINT('Ctrl Pts',(0.190321425282009,-0.0456338736779784,
-0.519808744594087));
#36466=CARTESIAN_POINT('Ctrl Pts',(0.205354381956416,0.0170628361432606,
-0.516116117704146));
#36467=CARTESIAN_POINT('Ctrl Pts',(0.186365665920766,0.0879170126515298,
-0.512423490814205));
#36468=CARTESIAN_POINT('Ctrl Pts',(0.141994204226371,0.134693508760327,
-0.508730863924265));
#36469=CARTESIAN_POINT('Ctrl Pts',(0.0976227425319756,0.181470004869124,
-0.505038237034324));
#36470=CARTESIAN_POINT('Ctrl Pts',(0.0278685351788353,0.204168820578448,
-0.501345610144383));
#36471=CARTESIAN_POINT('Ctrl Pts',(-0.0355337021850324,0.19246311688275,
-0.497652983254443));
#36472=CARTESIAN_POINT('Ctrl Pts',(-0.0989359395488994,0.180757413187051,
-0.493960356364502));
#36473=CARTESIAN_POINT('Ctrl Pts',(-0.155986206923494,0.134647190086329,
-0.49026772947456));
#36474=CARTESIAN_POINT('Ctrl Pts',(-0.180729453215574,0.0751103194393806,
-0.48657510258462));
#36475=CARTESIAN_POINT('Ctrl Pts',(-0.19053066592285,0.0515267715795701,
-0.485112391460554));
#36476=CARTESIAN_POINT('Ctrl Pts',(-0.195262634724071,0.0258364695538892,
-0.483649680336489));
#36477=CARTESIAN_POINT('Ctrl Pts',(-0.195139240617864,0.000102604098994689,
-0.482186969212423));
#36478=CARTESIAN_POINT('Origin',(0.,0.,-0.385));
#36479=CARTESIAN_POINT('',(-0.195293314183532,-0.000167834691889468,-0.402013030787577));
#36480=CARTESIAN_POINT('',(-0.195301750645145,-0.000169271322796084,-0.412186969212423));
#36481=CARTESIAN_POINT('',(-0.1954,-2.39295984553393E-17,-0.385));
#36482=CARTESIAN_POINT('Ctrl Pts',(-0.195293314183532,-0.000167834691889468,
-0.402013030787577));
#36483=CARTESIAN_POINT('Ctrl Pts',(-0.194911528013015,0.0458849723600842,
-0.404635882119527));
#36484=CARTESIAN_POINT('Ctrl Pts',(-0.178618575845566,0.0921809008404429,
-0.407258733451476));
#36485=CARTESIAN_POINT('Ctrl Pts',(-0.148897030686981,0.127021158074873,
-0.409881584783426));
#36486=CARTESIAN_POINT('Ctrl Pts',(-0.107053036127976,0.176071620504506,
-0.413574211673367));
#36487=CARTESIAN_POINT('Ctrl Pts',(-0.0385923533484633,0.202415904400708,
-0.417266838563308));
#36488=CARTESIAN_POINT('Ctrl Pts',(0.0253387916998359,0.194068663058447,
-0.420959465453248));
#36489=CARTESIAN_POINT('Ctrl Pts',(0.0892699367481351,0.185721421716186,
-0.424652092343189));
#36490=CARTESIAN_POINT('Ctrl Pts',(0.148671544065221,0.142682655135463,
-0.42834471923313));
#36491=CARTESIAN_POINT('Ctrl Pts',(0.176518819151958,0.0845328742635806,
-0.43203734612307));
#36492=CARTESIAN_POINT('Ctrl Pts',(0.204366094238696,0.0263830933916977,
-0.435729973013011));
#36493=CARTESIAN_POINT('Ctrl Pts',(0.200659037095084,-0.0468777017713445,
-0.439422599902952));
#36494=CARTESIAN_POINT('Ctrl Pts',(0.167084175443548,-0.101919471458649,
-0.443115226792893));
#36495=CARTESIAN_POINT('Ctrl Pts',(0.133509313792012,-0.156961241145953,
-0.446807853682834));
#36496=CARTESIAN_POINT('Ctrl Pts',(0.0700666476325517,-0.193783985357519,
-0.450500480572774));
#36497=CARTESIAN_POINT('Ctrl Pts',(0.00561945344688623,-0.195635176001563,
-0.454193107462715));
#36498=CARTESIAN_POINT('Ctrl Pts',(-0.0588277407387793,-0.197486366645606,
-0.457885734352656));
#36499=CARTESIAN_POINT('Ctrl Pts',(-0.12427946295065,-0.164366003722127,
-0.461578361242597));
#36500=CARTESIAN_POINT('Ctrl Pts',(-0.160958415531928,-0.11134221488443,
-0.465270988132538));
#36501=CARTESIAN_POINT('Ctrl Pts',(-0.1832813733445,-0.0790717240991829,
-0.467518335684218));
#36502=CARTESIAN_POINT('Ctrl Pts',(-0.194946930453413,-0.0394290272987776,
-0.469765683235897));
#36503=CARTESIAN_POINT('Ctrl Pts',(-0.195144246227183,0.000106621721020397,
-0.472013030787577));
#36504=CARTESIAN_POINT('Ctrl Pts',(-0.195139240617864,0.000102604098994689,
-0.482186969212423));
#36505=CARTESIAN_POINT('Ctrl Pts',(-0.194951125235189,-0.0391288964691331,
-0.479957053446548));
#36506=CARTESIAN_POINT('Ctrl Pts',(-0.1834785316021,-0.0784616439633596,
-0.477727137680673));
#36507=CARTESIAN_POINT('Ctrl Pts',(-0.161479272427984,-0.110585441722134,
-0.475497221914798));
#36508=CARTESIAN_POINT('Ctrl Pts',(-0.125049620138749,-0.163780814043522,
-0.471804595024857));
#36509=CARTESIAN_POINT('Ctrl Pts',(-0.0597540903507157,-0.197208040493121,
-0.468111968134916));
#36510=CARTESIAN_POINT('Ctrl Pts',(0.00470107911431957,-0.195659385673228,
-0.464419341244975));
#36511=CARTESIAN_POINT('Ctrl Pts',(0.0691562485793548,-0.194110730853336,
-0.460726714355034));
#36512=CARTESIAN_POINT('Ctrl Pts',(0.132771057721392,-0.157586194763953,
-0.457034087465094));
#36513=CARTESIAN_POINT('Ctrl Pts',(0.166603913510149,-0.10270263555075,
-0.453341460575153));
#36514=CARTESIAN_POINT('Ctrl Pts',(0.200436769298907,-0.0478190763375483,
-0.449648833685212));
#36515=CARTESIAN_POINT('Ctrl Pts',(0.204487671734386,0.0254235059994729,
-0.445956206795272));
#36516=CARTESIAN_POINT('Ctrl Pts',(0.176913660487352,0.0837033576319605,
-0.442263579905331));
#36517=CARTESIAN_POINT('Ctrl Pts',(0.149339649240319,0.141983209264448,
-0.43857095301539));
#36518=CARTESIAN_POINT('Ctrl Pts',(0.0901407243107727,0.185300330192403,
-0.434878326125449));
#36519=CARTESIAN_POINT('Ctrl Pts',(0.0262494697315635,0.193947572000777,
-0.431185699235508));
#36520=CARTESIAN_POINT('Ctrl Pts',(-0.0376417848476453,0.202594813809151,
-0.427493072345568));
#36521=CARTESIAN_POINT('Ctrl Pts',(-0.106225369076517,0.176572176497946,
-0.423800445455627));
#36522=CARTESIAN_POINT('Ctrl Pts',(-0.148299142919833,0.127718673479187,
-0.420107818565686));
#36523=CARTESIAN_POINT('Ctrl Pts',(-0.178382516650695,0.092787692606204,
-0.417467535447932));
#36524=CARTESIAN_POINT('Ctrl Pts',(-0.194912849038005,0.0461845170874172,
-0.414827252330178));
#36525=CARTESIAN_POINT('Ctrl Pts',(-0.195301750645145,-0.000169271322796084,
-0.412186969212423));
#36526=CARTESIAN_POINT('Origin',(0.,0.,-0.385));
#36527=CARTESIAN_POINT('',(-0.195708263869822,3.44180068116273E-5,-0.332013030787577));
#36528=CARTESIAN_POINT('',(-0.195705679436412,3.98752641654602E-5,-0.342186969212424));
#36529=CARTESIAN_POINT('',(-0.1954,-2.39295984553393E-17,-0.385));
#36530=CARTESIAN_POINT('Ctrl Pts',(-0.195708263869822,3.44180068116273E-5,
-0.332013030787577));
#36531=CARTESIAN_POINT('Ctrl Pts',(-0.195712867835684,0.0019167555331574,
-0.332120827223275));
#36532=CARTESIAN_POINT('Ctrl Pts',(-0.195688044184301,0.00379896863771164,
-0.332228623658972));
#36533=CARTESIAN_POINT('Ctrl Pts',(-0.195633418288648,0.00568031641885265,
-0.33233642009467));
#36534=CARTESIAN_POINT('Ctrl Pts',(-0.193762177835561,0.0701269315691545,
-0.336029046984611));
#36535=CARTESIAN_POINT('Ctrl Pts',(-0.156919698023893,0.133558138888658,
-0.339721673874551));
#36536=CARTESIAN_POINT('Ctrl Pts',(-0.101867485665295,0.167115875099989,
-0.343414300764492));
#36537=CARTESIAN_POINT('Ctrl Pts',(-0.0468152733066967,0.200673611311319,
-0.347106927654433));
#36538=CARTESIAN_POINT('Ctrl Pts',(0.026446671598832,0.204357876414479,
-0.350799554544373));
#36539=CARTESIAN_POINT('Ctrl Pts',(0.084587786207124,0.176492511939285,
-0.354492181434314));
#36540=CARTESIAN_POINT('Ctrl Pts',(0.142728900815417,0.14862714746409,-0.358184808324255));
#36541=CARTESIAN_POINT('Ctrl Pts',(0.185749185126472,0.089212153410541,
-0.361877435214196));
#36542=CARTESIAN_POINT('Ctrl Pts',(0.194076536712586,0.0252784145806732,
-0.365570062104137));
#36543=CARTESIAN_POINT('Ctrl Pts',(0.202403888298699,-0.0386553242491941,
-0.369262688994078));
#36544=CARTESIAN_POINT('Ctrl Pts',(0.17603830715987,-0.10710780785538,-0.372955315884018));
#36545=CARTESIAN_POINT('Ctrl Pts',(0.126974829193245,-0.148936540504495,
-0.376647942773959));
#36546=CARTESIAN_POINT('Ctrl Pts',(0.07791135122662,-0.19076527315361,-0.3803405696639));
#36547=CARTESIAN_POINT('Ctrl Pts',(0.00614997643219979,-0.205970254845654,
-0.384033196553841));
#36548=CARTESIAN_POINT('Ctrl Pts',(-0.0556614175584705,-0.187633970648876,
-0.387725823443782));
#36549=CARTESIAN_POINT('Ctrl Pts',(-0.117472811549142,-0.169297686452097,
-0.391418450333722));
#36550=CARTESIAN_POINT('Ctrl Pts',(-0.169334224736063,-0.117420136366495,
-0.395111077223663));
#36551=CARTESIAN_POINT('Ctrl Pts',(-0.187651278160274,-0.0556030408421606,
-0.398803704113603));
#36552=CARTESIAN_POINT('Ctrl Pts',(-0.192957835424703,-0.0376942675409406,
-0.399873479671594));
#36553=CARTESIAN_POINT('Ctrl Pts',(-0.195449032316932,-0.0189512734483915,
-0.400943255229586));
#36554=CARTESIAN_POINT('Ctrl Pts',(-0.195293314183532,-0.000167834691889468,
-0.402013030787577));
#36555=CARTESIAN_POINT('Ctrl Pts',(-0.195301750645145,-0.000169271322796084,
-0.412186969212423));
#36556=CARTESIAN_POINT('Ctrl Pts',(-0.195456756061615,-0.0186446083890101,
-0.411134625440237));
#36557=CARTESIAN_POINT('Ctrl Pts',(-0.193047535469114,-0.0370803278451861,
-0.41008228166805));
#36558=CARTESIAN_POINT('Ctrl Pts',(-0.187910199406209,-0.0547215890226383,
-0.409029937895864));
#36559=CARTESIAN_POINT('Ctrl Pts',(-0.169883518591507,-0.11662397977939,
-0.405337311005923));
#36560=CARTESIAN_POINT('Ctrl Pts',(-0.11826619350434,-0.168744392566579,
-0.401644684115982));
#36561=CARTESIAN_POINT('Ctrl Pts',(-0.0565415550860151,-0.187370616411795,
-0.397952057226041));
#36562=CARTESIAN_POINT('Ctrl Pts',(0.0051830833323095,-0.20599684025701,
-0.394259430336101));
#36563=CARTESIAN_POINT('Ctrl Pts',(0.0770150350817921,-0.191128875160252,
-0.39056680344616));
#36564=CARTESIAN_POINT('Ctrl Pts',(0.126274313505723,-0.149530910164822,
-0.386874176556219));
#36565=CARTESIAN_POINT('Ctrl Pts',(0.175533591929654,-0.107932945169391,
-0.383181549666278));
#36566=CARTESIAN_POINT('Ctrl Pts',(0.202220197028032,-0.0396049802752874,
-0.379488922776338));
#36567=CARTESIAN_POINT('Ctrl Pts',(0.194193042873466,0.0243671386421074,
-0.375796295886397));
#36568=CARTESIAN_POINT('Ctrl Pts',(0.1861658887189,0.0883392575595017,-0.372103668996456));
#36569=CARTESIAN_POINT('Ctrl Pts',(0.143424975311391,0.147955530500188,
-0.368411042106515));
#36570=CARTESIAN_POINT('Ctrl Pts',(0.0854153051300223,0.176093500719381,
-0.364718415216575));
#36571=CARTESIAN_POINT('Ctrl Pts',(0.0274056349486537,0.204231470938575,
-0.361025788326634));
#36572=CARTESIAN_POINT('Ctrl Pts',(-0.0458727920065736,0.200891138436277,
-0.357333161436693));
#36573=CARTESIAN_POINT('Ctrl Pts',(-0.101081914374396,0.167592189354063,
-0.353640534546752));
#36574=CARTESIAN_POINT('Ctrl Pts',(-0.156291036742218,0.134293240271849,
-0.349947907656811));
#36575=CARTESIAN_POINT('Ctrl Pts',(-0.193430854522634,0.0710356746097188,
-0.346255280766871));
#36576=CARTESIAN_POINT('Ctrl Pts',(-0.195604586827451,0.00659855727457022,
-0.34256265387693));
#36577=CARTESIAN_POINT('Ctrl Pts',(-0.195678304708696,0.00441329842142617,
-0.342437425655428));
#36578=CARTESIAN_POINT('Ctrl Pts',(-0.195711808283359,0.00222668297225595,
-0.342312197433926));
#36579=CARTESIAN_POINT('Ctrl Pts',(-0.195705679436412,3.98752641654602E-5,
-0.342186969212424));
#36580=CARTESIAN_POINT('Origin',(0.,0.,-0.385));
#36581=CARTESIAN_POINT('',(-0.19519881356068,0.000139152780809226,-0.262013030787577));
#36582=CARTESIAN_POINT('',(-0.195192130579109,0.000136023405943259,-0.272186969212423));
#36583=CARTESIAN_POINT('',(-0.1954,-2.39295984553393E-17,-0.385));
#36584=CARTESIAN_POINT('Ctrl Pts',(-0.19519881356068,0.000139152780809226,
-0.262013030787577));
#36585=CARTESIAN_POINT('Ctrl Pts',(-0.195348727543358,0.0227356530869617,
-0.263298399216963));
#36586=CARTESIAN_POINT('Ctrl Pts',(-0.191722703742678,0.0452855435778098,
-0.26458376764635));
#36587=CARTESIAN_POINT('Ctrl Pts',(-0.184108936130051,0.0663972888993632,
-0.265869136075736));
#36588=CARTESIAN_POINT('Ctrl Pts',(-0.162235983303931,0.127047447006306,
-0.269561762965677));
#36589=CARTESIAN_POINT('Ctrl Pts',(-0.107451896378664,0.175828490457768,
-0.273254389855617));
#36590=CARTESIAN_POINT('Ctrl Pts',(-0.0446807262998327,0.190547456158574,
-0.276947016745558));
#36591=CARTESIAN_POINT('Ctrl Pts',(0.0180904437789986,0.20526642185938,
-0.280639643635499));
#36592=CARTESIAN_POINT('Ctrl Pts',(0.0888486970113934,0.18592330980953,
-0.28433227052544));
#36593=CARTESIAN_POINT('Ctrl Pts',(0.135402526447063,0.141318279701041,
-0.288024897415381));
#36594=CARTESIAN_POINT('Ctrl Pts',(0.181956355882732,0.0967132495925533,
-0.291717524305321));
#36595=CARTESIAN_POINT('Ctrl Pts',(0.204305761521676,0.0268463014254276,
-0.295410151195262));
#36596=CARTESIAN_POINT('Ctrl Pts',(0.192282868776658,-0.0364965576431119,
-0.299102778085202));
#36597=CARTESIAN_POINT('Ctrl Pts',(0.18025997603164,-0.0998394167116532,
-0.302795404975143));
#36598=CARTESIAN_POINT('Ctrl Pts',(0.133864784902659,-0.156658186681608,
-0.306488031865084));
#36599=CARTESIAN_POINT('Ctrl Pts',(0.0742048135540952,-0.181103136340265,
-0.310180658755025));
#36600=CARTESIAN_POINT('Ctrl Pts',(0.0145448422055335,-0.205548085998922,
-0.313873285644966));
#36601=CARTESIAN_POINT('Ctrl Pts',(-0.058379909362609,-0.197619215346285,
-0.317565912534907));
#36602=CARTESIAN_POINT('Ctrl Pts',(-0.111392284599426,-0.160923768529416,
-0.321258539424847));
#36603=CARTESIAN_POINT('Ctrl Pts',(-0.162857104323945,-0.125299547831808,
-0.32484336987909));
#36604=CARTESIAN_POINT('Ctrl Pts',(-0.195555156423111,-0.0625637638898928,
-0.328428200333334));
#36605=CARTESIAN_POINT('Ctrl Pts',(-0.195708263869822,3.44180068116273E-5,
-0.332013030787577));
#36606=CARTESIAN_POINT('Ctrl Pts',(-0.195705679436412,3.98752641654602E-5,
-0.342186969212424));
#36607=CARTESIAN_POINT('Ctrl Pts',(-0.195531085880929,-0.0622561057247903,
-0.338619570543985));
#36608=CARTESIAN_POINT('Ctrl Pts',(-0.16319401629578,-0.124708108542943,
-0.335052171875546));
#36609=CARTESIAN_POINT('Ctrl Pts',(-0.112146426745488,-0.160399109455942,
-0.331484773207107));
#36610=CARTESIAN_POINT('Ctrl Pts',(-0.0593068875294896,-0.197342989843137,
-0.327792146317167));
#36611=CARTESIAN_POINT('Ctrl Pts',(0.0135798377317254,-0.205614081609361,
-0.324099519427226));
#36612=CARTESIAN_POINT('Ctrl Pts',(0.0733538925813345,-0.181449446924897,
-0.320406892537285));
#36613=CARTESIAN_POINT('Ctrl Pts',(0.133127947430945,-0.157284812240432,
-0.316714265647345));
#36614=CARTESIAN_POINT('Ctrl Pts',(0.179789331868949,-0.100684451105276,
-0.313021638757404));
#36615=CARTESIAN_POINT('Ctrl Pts',(0.19210942292752,-0.0373987295018618,
-0.309329011867463));
#36616=CARTESIAN_POINT('Ctrl Pts',(0.204429513986091,0.025886992101553,
-0.305636384977522));
#36617=CARTESIAN_POINT('Ctrl Pts',(0.18240831166523,0.0958580741732274,
-0.301943758087581));
#36618=CARTESIAN_POINT('Ctrl Pts',(0.136064374285097,0.140681133761328,
-0.298251131197641));
#36619=CARTESIAN_POINT('Ctrl Pts',(0.0897204369049655,0.185504193349427,
-0.2945585043077));
#36620=CARTESIAN_POINT('Ctrl Pts',(0.0190537644655635,0.205179230453953,
-0.290865877417759));
#36621=CARTESIAN_POINT('Ctrl Pts',(-0.0437858008467183,0.190755075924799,
-0.287173250527818));
#36622=CARTESIAN_POINT('Ctrl Pts',(-0.106625366159001,0.176330921395644,
-0.283480623637877));
#36623=CARTESIAN_POINT('Ctrl Pts',(-0.161637824344163,0.127807575232807,
-0.279787996747937));
#36624=CARTESIAN_POINT('Ctrl Pts',(-0.183795226765297,0.0672607609460622,
-0.276095369857996));
#36625=CARTESIAN_POINT('Ctrl Pts',(-0.191612607048412,0.045899165249305,
-0.274792569642805));
#36626=CARTESIAN_POINT('Ctrl Pts',(-0.195340329287759,0.0230409392171715,
-0.273489769427614));
#36627=CARTESIAN_POINT('Ctrl Pts',(-0.195192130579109,0.000136023405943259,
-0.272186969212423));
#36628=CARTESIAN_POINT('Origin',(0.,0.,-0.385));
#36629=CARTESIAN_POINT('',(-0.195221192409109,-0.000148384978497854,-0.192013030787577));
#36630=CARTESIAN_POINT('',(-0.195228501957461,-0.000151029643043509,-0.202186969212423));
#36631=CARTESIAN_POINT('',(-0.1954,-2.39295984553393E-17,-0.385));
#36632=CARTESIAN_POINT('Ctrl Pts',(-0.195221192409109,-0.000148384978497854,
-0.192013030787577));
#36633=CARTESIAN_POINT('Ctrl Pts',(-0.194912521452068,0.0431370728685057,
-0.194475971210652));
#36634=CARTESIAN_POINT('Ctrl Pts',(-0.18070219546031,0.0866065747243266,
-0.196938911633727));
#36635=CARTESIAN_POINT('Ctrl Pts',(-0.154226937755701,0.120493781946361,
-0.199401852056802));
#36636=CARTESIAN_POINT('Ctrl Pts',(-0.114533225474957,0.171300050518968,
-0.203094478946743));
#36637=CARTESIAN_POINT('Ctrl Pts',(-0.0472700584410176,0.200566970604116,
-0.206787105836683));
#36638=CARTESIAN_POINT('Ctrl Pts',(0.016961151042017,0.194979537104919,
-0.210479732726624));
#36639=CARTESIAN_POINT('Ctrl Pts',(0.0811923605250517,0.189392103605722,
-0.214172359616565));
#36640=CARTESIAN_POINT('Ctrl Pts',(0.142391612457181,0.148950316522181,
-0.217864986506506));
#36641=CARTESIAN_POINT('Ctrl Pts',(0.172716271241626,0.0920531913214624,
-0.221557613396447));
#36642=CARTESIAN_POINT('Ctrl Pts',(0.20304093002607,0.0351560661207439,
-0.225250240286387));
#36643=CARTESIAN_POINT('Ctrl Pts',(0.202490995662829,-0.0381963971971516,
-0.228942867176328));
#36644=CARTESIAN_POINT('Ctrl Pts',(0.17131666197679,-0.0946324553291228,
-0.232635494066269));
#36645=CARTESIAN_POINT('Ctrl Pts',(0.140142328290751,-0.151068513461093,
-0.236328120956209));
#36646=CARTESIAN_POINT('Ctrl Pts',(0.0783435952819142,-0.19058816640714,
-0.24002074784615));
#36647=CARTESIAN_POINT('Ctrl Pts',(0.0140358306636315,-0.195211925443371,
-0.243713374736091));
#36648=CARTESIAN_POINT('Ctrl Pts',(-0.0502719339546524,-0.199835684479602,
-0.247406001626032));
#36649=CARTESIAN_POINT('Ctrl Pts',(-0.117088730182383,-0.169563549606015,
-0.251098628515973));
#36650=CARTESIAN_POINT('Ctrl Pts',(-0.156016218932762,-0.11816784578801,
-0.254791255405913));
#36651=CARTESIAN_POINT('Ctrl Pts',(-0.181393417722536,-0.0846624994479597,
-0.257198513866468));
#36652=CARTESIAN_POINT('Ctrl Pts',(-0.194918052266947,-0.042179932780427,
-0.259605772327022));
#36653=CARTESIAN_POINT('Ctrl Pts',(-0.19519881356068,0.000139152780809226,
-0.262013030787577));
#36654=CARTESIAN_POINT('Ctrl Pts',(-0.195192130579109,0.000136023405943259,
-0.272186969212423));
#36655=CARTESIAN_POINT('Ctrl Pts',(-0.19492027828513,-0.0418802260161198,
-0.269797142537674));
#36656=CARTESIAN_POINT('Ctrl Pts',(-0.181606189342149,-0.0840535836858002,
-0.267407315862924));
#36657=CARTESIAN_POINT('Ctrl Pts',(-0.156569170098022,-0.117434195704244,
-0.265017489188174));
#36658=CARTESIAN_POINT('Ctrl Pts',(-0.117883364352505,-0.169012055657157,
-0.261324862298233));
#36659=CARTESIAN_POINT('Ctrl Pts',(-0.051209406204363,-0.19959749315233,
-0.257632235408292));
#36660=CARTESIAN_POINT('Ctrl Pts',(0.0131193497373221,-0.195275646237997,
-0.253939608518351));
#36661=CARTESIAN_POINT('Ctrl Pts',(0.0774481056790059,-0.190953799323664,
-0.25024698162841));
#36662=CARTESIAN_POINT('Ctrl Pts',(0.139431659414233,-0.151724667999826,
-0.24655435473847));
#36663=CARTESIAN_POINT('Ctrl Pts',(0.170870558530041,-0.0954355676028622,
-0.242861727848529));
#36664=CARTESIAN_POINT('Ctrl Pts',(0.202309457645848,-0.0391464672058984,
-0.239169100958588));
#36665=CARTESIAN_POINT('Ctrl Pts',(0.203203702142237,0.0342026022641913,
-0.235476474068647));
#36666=CARTESIAN_POINT('Ctrl Pts',(0.17314645488136,0.091241440750627,-0.231783847178707));
#36667=CARTESIAN_POINT('Ctrl Pts',(0.143089207620483,0.148280279237063,
-0.228091220288766));
#36668=CARTESIAN_POINT('Ctrl Pts',(0.0820804686023399,0.189008886739845,
-0.224398593398825));
#36669=CARTESIAN_POINT('Ctrl Pts',(0.0178761979905637,0.194897760180302,
-0.220705966508884));
#36670=CARTESIAN_POINT('Ctrl Pts',(-0.0463280726212126,0.200786633620759,
-0.217013339618944));
#36671=CARTESIAN_POINT('Ctrl Pts',(-0.113727874826622,0.171835772998892,
-0.213320712729003));
#36672=CARTESIAN_POINT('Ctrl Pts',(-0.153659631261092,0.121216389126229,
-0.209628085839062));
#36673=CARTESIAN_POINT('Ctrl Pts',(-0.180482167591968,0.0872148729344941,
-0.207147713630182));
#36674=CARTESIAN_POINT('Ctrl Pts',(-0.194911299555516,0.0434366593785047,
-0.204667341421303));
#36675=CARTESIAN_POINT('Ctrl Pts',(-0.195228501957461,-0.000151029643043509,
-0.202186969212423));
#36676=CARTESIAN_POINT('Origin',(0.,0.,-0.385));
#36677=CARTESIAN_POINT('',(-0.195714129816575,-1.66459635889404E-5,-0.122013030787577));
#36678=CARTESIAN_POINT('',(-0.195715049123435,-1.11371353569391E-5,-0.132186969212423));
#36679=CARTESIAN_POINT('',(-0.1954,-2.39295984553393E-17,-0.385));
#36680=CARTESIAN_POINT('Ctrl Pts',(-0.195714129816575,-1.66459635889404E-5,
-0.122013030787577));
#36681=CARTESIAN_POINT('Ctrl Pts',(-0.19563573648805,0.0635488758200351,
-0.125653543204341));
#36682=CARTESIAN_POINT('Ctrl Pts',(-0.161767712733412,0.127185954073863,
-0.129294055621104));
#36683=CARTESIAN_POINT('Ctrl Pts',(-0.10896691742764,0.162575785310205,
-0.132934568037868));
#36684=CARTESIAN_POINT('Ctrl Pts',(-0.0554102709350894,0.198472227209985,
-0.136627194927809));
#36685=CARTESIAN_POINT('Ctrl Pts',(0.0176250777221782,0.205306906538936,
-0.140319821817749));
#36686=CARTESIAN_POINT('Ctrl Pts',(0.0769118082973,0.179970218457928,-0.14401244870769));
#36687=CARTESIAN_POINT('Ctrl Pts',(0.136198538872421,0.15463353037692,-0.147705075597631));
#36688=CARTESIAN_POINT('Ctrl Pts',(0.181736651365396,0.0971254748859523,
-0.151397702487572));
#36689=CARTESIAN_POINT('Ctrl Pts',(0.192808475960345,0.0336094599183851,
-0.155090329377513));
#36690=CARTESIAN_POINT('Ctrl Pts',(0.203880300555293,-0.0299065550491812,
-0.158782956267453));
#36691=CARTESIAN_POINT('Ctrl Pts',(0.180485837252216,-0.0994305294933474,
-0.162475583157394));
#36692=CARTESIAN_POINT('Ctrl Pts',(0.133268452240781,-0.1433325374099,-0.166168210047335));
#36693=CARTESIAN_POINT('Ctrl Pts',(0.0860510672293448,-0.187234545326454,
-0.169860836937276));
#36694=CARTESIAN_POINT('Ctrl Pts',(0.0150107605095506,-0.205514586715394,
-0.173553463827216));
#36695=CARTESIAN_POINT('Ctrl Pts',(-0.0475326626638961,-0.189856122850204,
-0.177246090717157));
#36696=CARTESIAN_POINT('Ctrl Pts',(-0.110076085837342,-0.174197658985015,
-0.180938717607098));
#36697=CARTESIAN_POINT('Ctrl Pts',(-0.164122625464441,-0.124600689865696,
-0.184631344497039));
#36698=CARTESIAN_POINT('Ctrl Pts',(-0.185083766514216,-0.0636293967760041,
-0.188323971386979));
#36699=CARTESIAN_POINT('Ctrl Pts',(-0.192064063264259,-0.0433252674354672,
-0.189553657853845));
#36700=CARTESIAN_POINT('Ctrl Pts',(-0.195375304337693,-0.0217597651109067,
-0.190783344320711));
#36701=CARTESIAN_POINT('Ctrl Pts',(-0.195221192409109,-0.000148384978497854,
-0.192013030787577));
#36702=CARTESIAN_POINT('Ctrl Pts',(-0.195228501957461,-0.000151029643043509,
-0.202186969212423));
#36703=CARTESIAN_POINT('Ctrl Pts',(-0.195383531148332,-0.0214540340324061,
-0.200974714531362));
#36704=CARTESIAN_POINT('Ctrl Pts',(-0.192167702584793,-0.0427115286208927,
-0.199762459850301));
#36705=CARTESIAN_POINT('Ctrl Pts',(-0.185380390392341,-0.0627599095134647,
-0.19855020516924));
#36706=CARTESIAN_POINT('Ctrl Pts',(-0.164705682425589,-0.123828917157039,
-0.194857578279299));
#36707=CARTESIAN_POINT('Ctrl Pts',(-0.110892555828552,-0.173679025320728,
-0.191164951389358));
#36708=CARTESIAN_POINT('Ctrl Pts',(-0.0484233240331688,-0.189630897337212,
-0.187472324499417));
#36709=CARTESIAN_POINT('Ctrl Pts',(0.0140459077622141,-0.205582769353695,
-0.183779697609477));
#36710=CARTESIAN_POINT('Ctrl Pts',(0.0851712447559427,-0.187636405222974,
-0.180087070719536));
#36711=CARTESIAN_POINT('Ctrl Pts',(0.132594177669105,-0.14395651726514,
-0.176394443829595));
#36712=CARTESIAN_POINT('Ctrl Pts',(0.180017110582266,-0.100276629307306,
-0.172701816939654));
#36713=CARTESIAN_POINT('Ctrl Pts',(0.203737639414863,-0.0308632175223595,
-0.169009190049713));
#36714=CARTESIAN_POINT('Ctrl Pts',(0.192964091346187,0.0327040549976082,
-0.165316563159773));
#36715=CARTESIAN_POINT('Ctrl Pts',(0.182190543277511,0.0962713275175769,
-0.161623936269832));
#36716=CARTESIAN_POINT('Ctrl Pts',(0.136922918307562,0.153992460772567,
-0.157931309379891));
#36717=CARTESIAN_POINT('Ctrl Pts',(0.0777557571850433,0.179607178680573,
-0.15423868248995));
#36718=CARTESIAN_POINT('Ctrl Pts',(0.0185885960625246,0.205221896588578,
-0.15054605560001));
#36719=CARTESIAN_POINT('Ctrl Pts',(-0.0544781012125634,0.198730199149599,
-0.146853428710069));
#36720=CARTESIAN_POINT('Ctrl Pts',(-0.108202617777375,0.163085514791286,
-0.143160801820128));
#36721=CARTESIAN_POINT('Ctrl Pts',(-0.161422531340639,0.127775620131725,
-0.13950285761756));
#36722=CARTESIAN_POINT('Ctrl Pts',(-0.195661897485078,0.0638578007034306,
-0.135844913414992));
#36723=CARTESIAN_POINT('Ctrl Pts',(-0.195715049123435,-1.11371353569391E-5,
-0.132186969212423));
#36724=CARTESIAN_POINT('Origin',(0.,0.,-0.385));
#36725=CARTESIAN_POINT('',(-0.195265563427387,0.000160747932399612,-0.0520130307875765));
#36726=CARTESIAN_POINT('',(-0.195258838497135,0.000160033407109407,-0.0621869692124234));
#36727=CARTESIAN_POINT('',(-0.1954,-2.39295984553393E-17,-0.385));
#36728=CARTESIAN_POINT('Ctrl Pts',(-0.195265563427387,0.000160747932399612,
-0.0520130307875765));
#36729=CARTESIAN_POINT('Ctrl Pts',(-0.195424699897344,0.0199310521824771,
-0.0531384883080881));
#36730=CARTESIAN_POINT('Ctrl Pts',(-0.192664102409213,0.0396584116229354,
-0.0542639458285998));
#36731=CARTESIAN_POINT('Ctrl Pts',(-0.186800565614977,0.0584146868577315,
-0.0553894033491114));
#36732=CARTESIAN_POINT('Ctrl Pts',(-0.167562297406761,0.119954038654549,
-0.0590820302390522));
#36733=CARTESIAN_POINT('Ctrl Pts',(-0.114920994740183,0.171039702517518,
-0.0627746571289931));
#36734=CARTESIAN_POINT('Ctrl Pts',(-0.0528397488128431,0.188445146666394,
-0.066467284018934));
#36735=CARTESIAN_POINT('Ctrl Pts',(0.00924149711449647,0.205850590815268,
-0.0701599109088748));
#36736=CARTESIAN_POINT('Ctrl Pts',(0.0807626863026003,0.189575815250048,
-0.0738525377988157));
#36737=CARTESIAN_POINT('Ctrl Pts',(0.129192507975583,0.147017210543397,
-0.0775451646887565));
#36738=CARTESIAN_POINT('Ctrl Pts',(0.177622329648565,0.104458605836747,
-0.0812377915786972));
#36739=CARTESIAN_POINT('Ctrl Pts',(0.202960783806429,0.0356161719886669,
-0.0849304184686379));
#36740=CARTESIAN_POINT('Ctrl Pts',(0.193676298191635,-0.0281860789989965,
-0.0886230453585787));
#36741=CARTESIAN_POINT('Ctrl Pts',(0.18439181257684,-0.0919883299866607,
-0.0923156722485195));
#36742=CARTESIAN_POINT('Ctrl Pts',(0.140484387189387,-0.150750398113907,
-0.0960082991384602));
#36743=CARTESIAN_POINT('Ctrl Pts',(0.081931739171364,-0.177740603840422,
-0.099700926028401));
#36744=CARTESIAN_POINT('Ctrl Pts',(0.0233790911533422,-0.204730809566937,
-0.103393552918342));
#36745=CARTESIAN_POINT('Ctrl Pts',(-0.0498187794952493,-0.199949152892722,
-0.107086179808282));
#36746=CARTESIAN_POINT('Ctrl Pts',(-0.104361515224881,-0.165569919440996,
-0.110778806698223));
#36747=CARTESIAN_POINT('Ctrl Pts',(-0.158904250954513,-0.131190685989269,
-0.114471433588164));
#36748=CARTESIAN_POINT('Ctrl Pts',(-0.194791851765185,-0.0672138757600308,
-0.118164060478105));
#36749=CARTESIAN_POINT('Ctrl Pts',(-0.195696680006605,-0.00274636841010696,
-0.121856687368046));
#36750=CARTESIAN_POINT('Ctrl Pts',(-0.195709449952912,-0.00183653097385362,
-0.121908801841223));
#36751=CARTESIAN_POINT('Ctrl Pts',(-0.195715252028656,-0.000926595800520846,
-0.1219609163144));
#36752=CARTESIAN_POINT('Ctrl Pts',(-0.195714129816575,-1.66459635889404E-5,
-0.122013030787577));
#36753=CARTESIAN_POINT('Ctrl Pts',(-0.195715049123435,-1.11371353569391E-5,
-0.132186969212423));
#36754=CARTESIAN_POINT('Ctrl Pts',(-0.195715553079087,-0.000616708538638704,
-0.132152286525051));
#36755=CARTESIAN_POINT('Ctrl Pts',(-0.195712983753233,-0.00122227554755018,
-0.132117603837678));
#36756=CARTESIAN_POINT('Ctrl Pts',(-0.195707328185051,-0.00182781373595469,
-0.132082921150306));
#36757=CARTESIAN_POINT('Ctrl Pts',(-0.195105186173382,-0.0662987866272353,
-0.128390294260365));
#36758=CARTESIAN_POINT('Ctrl Pts',(-0.159518566295507,-0.130443061132149,
-0.124697667370424));
#36759=CARTESIAN_POINT('Ctrl Pts',(-0.105137686353204,-0.165078065539304,
-0.121005040480483));
#36760=CARTESIAN_POINT('Ctrl Pts',(-0.0507568064109017,-0.199713069946459,
-0.117312413590543));
#36761=CARTESIAN_POINT('Ctrl Pts',(0.0224183335958285,-0.204838804255855,
-0.113619786700602));
#36762=CARTESIAN_POINT('Ctrl Pts',(0.0810967868923935,-0.178123499671584,
-0.109927159810661));
#36763=CARTESIAN_POINT('Ctrl Pts',(0.139775240188958,-0.151408195087312,
-0.10623453292072));
#36764=CARTESIAN_POINT('Ctrl Pts',(0.183957006775358,-0.0928518516093715,
-0.10254190603078));
#36765=CARTESIAN_POINT('Ctrl Pts',(0.193541330769425,-0.0290943544827345,
-0.0988492791408388));
#36766=CARTESIAN_POINT('Ctrl Pts',(0.203125654763491,0.034663142643903,
-0.095156652250898));
#36767=CARTESIAN_POINT('Ctrl Pts',(0.178112536165224,0.103621793419236,
-0.0914640253609573));
#36768=CARTESIAN_POINT('Ctrl Pts',(0.129882157652608,0.14640814297767,-0.0877713984710165));
#36769=CARTESIAN_POINT('Ctrl Pts',(0.0816517791399922,0.189194492536102,
-0.0840787715810758));
#36770=CARTESIAN_POINT('Ctrl Pts',(0.0102041407130279,0.205808540877635,
-0.0803861446911351));
#36771=CARTESIAN_POINT('Ctrl Pts',(-0.0519564723881836,0.188693009030546,
-0.0766935178011943));
#36772=CARTESIAN_POINT('Ctrl Pts',(-0.114117085489396,0.171577477183457,
-0.0730008909112535));
#36773=CARTESIAN_POINT('Ctrl Pts',(-0.166990673264856,0.120732365147745,
-0.0693082640213127));
#36774=CARTESIAN_POINT('Ctrl Pts',(-0.1865207333334,0.059287224845946,-0.0656156371313719));
#36775=CARTESIAN_POINT('Ctrl Pts',(-0.192565399493649,0.0402695997597707,
-0.0644727478250558));
#36776=CARTESIAN_POINT('Ctrl Pts',(-0.195415961833315,0.0202365574963669,
-0.0633298585187396));
#36777=CARTESIAN_POINT('Ctrl Pts',(-0.195258838497135,0.000160033407109407,
-0.0621869692124234));
#36778=CARTESIAN_POINT('Origin',(0.,0.,-0.90400562256037));
#36779=CARTESIAN_POINT('',(-0.155442980507318,0.000127964897052157,-0.0290056225603697));
#36780=CARTESIAN_POINT('',(-0.155327760552453,-0.000155038459510079,-0.0151943774396293));
#36781=CARTESIAN_POINT('',(-0.15555,-8.39731161192283E-15,-0.90400562256037));
#36782=CARTESIAN_POINT('',(0.133815347598873,-0.0797905857758447,1.38777878078145E-16));
#36783=CARTESIAN_POINT('Ctrl Pts',(-0.155442980507318,0.000127964897052158,
-0.0290056225603697));
#36784=CARTESIAN_POINT('Ctrl Pts',(-0.155154018602902,-0.035771189888286,
-0.0264384531909407));
#36785=CARTESIAN_POINT('Ctrl Pts',(-0.124961417838318,-0.123741558504079,
-0.0201786569315709));
#36786=CARTESIAN_POINT('Ctrl Pts',(0.0168354762982751,-0.18072128944305,
-0.0105101160781143));
#36787=CARTESIAN_POINT('Ctrl Pts',(0.109303704153288,-0.120379820697564,
-0.00340874459408667));
#36788=CARTESIAN_POINT('Ctrl Pts',(0.133815347598873,-0.0797905857758447,
1.25821662116943E-16));
#36789=CARTESIAN_POINT('',(-0.0319621170202007,-0.152230829911641,0.));
#36790=CARTESIAN_POINT('Origin',(0.,0.,1.11022302462516E-16));
#36791=CARTESIAN_POINT('Ctrl Pts',(-0.155327760552453,-0.000155038459510074,
-0.0151943774396293));
#36792=CARTESIAN_POINT('Ctrl Pts',(-0.155432057916671,-0.0193751812911555,
-0.0138222118496936));
#36793=CARTESIAN_POINT('Ctrl Pts',(-0.143247305876585,-0.090139499299076,
-0.00875741936981715));
#36794=CARTESIAN_POINT('Ctrl Pts',(-0.0824189364736414,-0.141637004936936,
-0.00369262688994078));
#36795=CARTESIAN_POINT('Ctrl Pts',(-0.0319621170202007,-0.152230829911641,
0.));
#36796=CARTESIAN_POINT('Origin',(0.,0.,-0.90400562256037));
#36797=CARTESIAN_POINT('',(-0.155800065982437,-1.32511752194797E-5,-0.0990056225603699));
#36798=CARTESIAN_POINT('',(-0.15543762706361,0.000127396092498608,-0.0851943774396296));
#36799=CARTESIAN_POINT('',(-0.15555,-8.39731161192283E-15,-0.90400562256037));
#36800=CARTESIAN_POINT('Ctrl Pts',(-0.155800065982437,-1.32511752195067E-5,
-0.0990056225603699));
#36801=CARTESIAN_POINT('Ctrl Pts',(-0.155800959329875,-0.00073762526495506,
-0.0989535080871929));
#36802=CARTESIAN_POINT('Ctrl Pts',(-0.155469070736801,-0.0527874635943024,
-0.0952087667240751));
#36803=CARTESIAN_POINT('Ctrl Pts',(-0.0979285564476671,-0.155364913187252,
-0.0877713984710165));
#36804=CARTESIAN_POINT('Ctrl Pts',(0.0768809949247246,-0.16678436092022,
-0.0766935178011943));
#36805=CARTESIAN_POINT('Ctrl Pts',(0.181739746496141,-0.0264500769305604,
-0.0656156371313721));
#36806=CARTESIAN_POINT('Ctrl Pts',(0.121227005284432,0.137957915675413,
-0.0545377564615496));
#36807=CARTESIAN_POINT('Ctrl Pts',(-0.0495783321496912,0.176824978201047,
-0.0434598757917274));
#36808=CARTESIAN_POINT('Ctrl Pts',(-0.146161737697263,0.0830957743134539,
-0.034949164491334));
#36809=CARTESIAN_POINT('Ctrl Pts',(-0.155569662584605,0.0158663007522202,
-0.0301310800808815));
#36810=CARTESIAN_POINT('Ctrl Pts',(-0.155442980507318,0.000127964897052158,
-0.0290056225603697));
#36811=CARTESIAN_POINT('Ctrl Pts',(-0.15543762706361,0.000127396092498587,
-0.0851943774396296));
#36812=CARTESIAN_POINT('Ctrl Pts',(-0.155158579995167,-0.0355280025756548,
-0.0826446398560051));
#36813=CARTESIAN_POINT('Ctrl Pts',(-0.125300184105867,-0.123242688352141,
-0.0764022753824399));
#36814=CARTESIAN_POINT('Ctrl Pts',(0.0201819892413759,-0.182531533674816,
-0.0664672840189338));
#36815=CARTESIAN_POINT('Ctrl Pts',(0.164054917332699,-0.0825830908935778,
-0.0553894033491116));
#36816=CARTESIAN_POINT('Ctrl Pts',(0.158618708021993,0.0925610883157775,
-0.0443115226792891));
#36817=CARTESIAN_POINT('Ctrl Pts',(0.00892266599271826,0.183382072237952,
-0.0332336420094669));
#36818=CARTESIAN_POINT('Ctrl Pts',(-0.129457814449668,0.116933784740767,
-0.0235279269295804));
#36819=CARTESIAN_POINT('Ctrl Pts',(-0.155151383882512,0.0323480340184218,
-0.0175148387396345));
#36820=CARTESIAN_POINT('Ctrl Pts',(-0.155327760552453,-0.000155038459510074,
-0.0151943774396293));
#36821=CARTESIAN_POINT('Origin',(0.,0.,-0.90400562256037));
#36822=CARTESIAN_POINT('',(-0.155407658542666,-0.000118123251820218,-0.16900562256037));
#36823=CARTESIAN_POINT('',(-0.155800797805273,-8.86582091297328E-6,-0.15519437743963));
#36824=CARTESIAN_POINT('',(-0.15555,-8.39731161192283E-15,-0.90400562256037));
#36825=CARTESIAN_POINT('Ctrl Pts',(-0.155407658542666,-0.00011812325182025,
-0.16900562256037));
#36826=CARTESIAN_POINT('Ctrl Pts',(-0.155530340786735,-0.0173220648055368,
-0.167775936093504));
#36827=CARTESIAN_POINT('Ctrl Pts',(-0.144978915679302,-0.086041550229714,
-0.162853622736698));
#36828=CARTESIAN_POINT('Ctrl Pts',(-0.044602845000016,-0.178153809629627,
-0.15423868248995));
#36829=CARTESIAN_POINT('Ctrl Pts',(0.125054059456442,-0.134497815186694,
-0.143160801820128));
#36830=CARTESIAN_POINT('Ctrl Pts',(0.180924204289506,0.0315378177425299,
-0.132082921150306));
#36831=CARTESIAN_POINT('Ctrl Pts',(0.0721710814909035,0.168877296221853,
-0.121005040480484));
#36832=CARTESIAN_POINT('Ctrl Pts',(-0.101429795153458,0.152631651545641,
-0.109979274283838));
#36833=CARTESIAN_POINT('Ctrl Pts',(-0.155737660239083,0.0505886777574477,
-0.102646134977134));
#36834=CARTESIAN_POINT('Ctrl Pts',(-0.155800065982437,-1.32511752195067E-5,
-0.0990056225603699));
#36835=CARTESIAN_POINT('Ctrl Pts',(-0.155800797805273,-8.86582091298835E-6,
-0.15519437743963));
#36836=CARTESIAN_POINT('Ctrl Pts',(-0.15580119898389,-0.000490936607914258,
-0.155159694752257));
#36837=CARTESIAN_POINT('Ctrl Pts',(-0.155581389023891,-0.052298168361465,
-0.151432385174944));
#36838=CARTESIAN_POINT('Ctrl Pts',(-0.0986571866185378,-0.154903070922954,
-0.14401244870769));
#36839=CARTESIAN_POINT('Ctrl Pts',(0.0760980799328472,-0.16714423732766,
-0.132934568037868));
#36840=CARTESIAN_POINT('Ctrl Pts',(0.181612007146477,-0.027301260439323,
-0.121856687368045));
#36841=CARTESIAN_POINT('Ctrl Pts',(0.121876225192118,0.137384278886722,
-0.110778806698223));
#36842=CARTESIAN_POINT('Ctrl Pts',(-0.0487534599252984,0.177061585225392,
-0.0997009260284008));
#36843=CARTESIAN_POINT('Ctrl Pts',(-0.145961746301879,0.0835826589870833,
-0.091172782942203));
#36844=CARTESIAN_POINT('Ctrl Pts',(-0.1555627065669,0.0161095011185192,
-0.0863372667459459));
#36845=CARTESIAN_POINT('Ctrl Pts',(-0.15543762706361,0.000127396092498587,
-0.0851943774396296));
#36846=CARTESIAN_POINT('Origin',(0.,0.,-0.90400562256037));
#36847=CARTESIAN_POINT('',(-0.155389843650787,0.000110773874380199,-0.23900562256037));
#36848=CARTESIAN_POINT('',(-0.155413477377088,-0.000120228561807947,-0.22519437743963));
#36849=CARTESIAN_POINT('',(-0.15555,-8.39731161192283E-15,-0.90400562256037));
#36850=CARTESIAN_POINT('Ctrl Pts',(-0.155389843650787,0.000110773874380203,
-0.23900562256037));
#36851=CARTESIAN_POINT('Ctrl Pts',(-0.155166340993467,-0.0335777305219866,
-0.236598364099816));
#36852=CARTESIAN_POINT('Ctrl Pts',(-0.127884734191329,-0.119272665639336,
-0.23049847874932));
#36853=CARTESIAN_POINT('Ctrl Pts',(0.0131706925618085,-0.183179484648865,
-0.220705966508885));
#36854=CARTESIAN_POINT('Ctrl Pts',(0.160757073107222,-0.0887995151131783,
-0.209628085839062));
#36855=CARTESIAN_POINT('Ctrl Pts',(0.162070414307866,0.0863792310858789,
-0.19855020516924));
#36856=CARTESIAN_POINT('Ctrl Pts',(0.0159157013389389,0.182961421170497,
-0.187472324499417));
#36857=CARTESIAN_POINT('Ctrl Pts',(-0.126889473131666,0.12082536940136,
-0.177624130296461));
#36858=CARTESIAN_POINT('Ctrl Pts',(-0.155161938136486,0.0343396708530999,
-0.171468562983445));
#36859=CARTESIAN_POINT('Ctrl Pts',(-0.155407658542666,-0.00011812325182025,
-0.16900562256037));
#36860=CARTESIAN_POINT('Ctrl Pts',(-0.155413477377088,-0.000120228561807949,
-0.22519437743963));
#36861=CARTESIAN_POINT('Ctrl Pts',(-0.155536889816391,-0.0170786847172067,
-0.223982122758568));
#36862=CARTESIAN_POINT('Ctrl Pts',(-0.14517895913199,-0.0855474016034071,
-0.219077241187567));
#36863=CARTESIAN_POINT('Ctrl Pts',(-0.045438614211677,-0.177942460150977,
-0.210479732726624));
#36864=CARTESIAN_POINT('Ctrl Pts',(0.124421357682504,-0.135083346427328,
-0.199401852056802));
#36865=CARTESIAN_POINT('Ctrl Pts',(0.181070205071097,0.0306882431808897,
-0.18832397138698));
#36866=CARTESIAN_POINT('Ctrl Pts',(0.0729630546502829,0.168536589309041,
-0.177246090717157));
#36867=CARTESIAN_POINT('Ctrl Pts',(-0.100986917449906,0.153081797584407,
-0.166202892734707));
#36868=CARTESIAN_POINT('Ctrl Pts',(-0.155758485945775,0.050834600304081,
-0.158852321642198));
#36869=CARTESIAN_POINT('Ctrl Pts',(-0.155800797805273,-8.86582091298835E-6,
-0.15519437743963));
#36870=CARTESIAN_POINT('Origin',(0.,0.,-0.90400562256037));
#36871=CARTESIAN_POINT('',(-0.155795396340587,2.73987766570263E-5,-0.30900562256037));
#36872=CARTESIAN_POINT('',(-0.155384523600718,0.000108282706206955,-0.29519437743963));
#36873=CARTESIAN_POINT('',(-0.15555,-8.39731161192283E-15,-0.90400562256037));
#36874=CARTESIAN_POINT('Ctrl Pts',(-0.155795396340587,2.73987766570313E-5,
-0.30900562256037));
#36875=CARTESIAN_POINT('Ctrl Pts',(-0.155673513723719,-0.0498044701794957,
-0.305420792106127));
#36876=CARTESIAN_POINT('Ctrl Pts',(-0.102831618486219,-0.151189033169581,
-0.298143334761943));
#36877=CARTESIAN_POINT('Ctrl Pts',(0.0696309893116479,-0.169940330640481,
-0.287173250527819));
#36878=CARTESIAN_POINT('Ctrl Pts',(0.180430968535489,-0.0342469887444786,
-0.276095369857996));
#36879=CARTESIAN_POINT('Ctrl Pts',(0.127056607525184,0.132607726517495,
-0.265017489188174));
#36880=CARTESIAN_POINT('Ctrl Pts',(-0.0419267029707069,0.178802523027537,
-0.253939608518351));
#36881=CARTESIAN_POINT('Ctrl Pts',(-0.144330183939881,0.0876200476939117,
-0.245268986309084));
#36882=CARTESIAN_POINT('Ctrl Pts',(-0.155509184080703,0.0180989295684548,
-0.240290990989756));
#36883=CARTESIAN_POINT('Ctrl Pts',(-0.155389843650787,0.000110773874380203,
-0.23900562256037));
#36884=CARTESIAN_POINT('Ctrl Pts',(-0.155384523600718,0.000108282706206955,
-0.29519437743963));
#36885=CARTESIAN_POINT('Ctrl Pts',(-0.155168113036088,-0.0333391461453875,
-0.29280455076488));
#36886=CARTESIAN_POINT('Ctrl Pts',(-0.128192625181579,-0.118785991398888,
-0.286722097200189));
#36887=CARTESIAN_POINT('Ctrl Pts',(0.0123107014066272,-0.183239277698152,
-0.276947016745558));
#36888=CARTESIAN_POINT('Ctrl Pts',(0.160338466762532,-0.0895531255371017,
-0.265869136075736));
#36889=CARTESIAN_POINT('Ctrl Pts',(0.162474081881463,0.0856175155489654,
-0.254791255405913));
#36890=CARTESIAN_POINT('Ctrl Pts',(0.0167743476807649,0.182884683876359,
-0.243713374736091));
#36891=CARTESIAN_POINT('Ctrl Pts',(-0.126574199990401,0.121310855939487,
-0.23384774874733));
#36892=CARTESIAN_POINT('Ctrl Pts',(-0.155160965434293,0.0345781595001282,
-0.227674749648509));
#36893=CARTESIAN_POINT('Ctrl Pts',(-0.155413477377088,-0.000120228561807949,
-0.22519437743963));
#36894=CARTESIAN_POINT('Origin',(0.,0.,-0.90400562256037));
#36895=CARTESIAN_POINT('',(-0.155465071756645,-0.000133606378324517,-0.37900562256037));
#36896=CARTESIAN_POINT('',(-0.155793338978167,3.17430774774384E-5,-0.36519437743963));
#36897=CARTESIAN_POINT('',(-0.15555,-8.39731161192283E-15,-0.90400562256037));
#36898=CARTESIAN_POINT('Ctrl Pts',(-0.155465071756645,-0.000133606378324543,
-0.37900562256037));
#36899=CARTESIAN_POINT('Ctrl Pts',(-0.155589032635101,-0.0150863387149346,
-0.377935847002379));
#36900=CARTESIAN_POINT('Ctrl Pts',(-0.146760532433313,-0.0815092407522182,
-0.373173444554447));
#36901=CARTESIAN_POINT('Ctrl Pts',(-0.0522305681435164,-0.176068618441347,
-0.364718415216575));
#36902=CARTESIAN_POINT('Ctrl Pts',(0.119148375294644,-0.139756414211085,
-0.353640534546752));
#36903=CARTESIAN_POINT('Ctrl Pts',(0.182114078664316,0.023720307768581,
-0.34256265387693));
#36904=CARTESIAN_POINT('Ctrl Pts',(0.0793739779798006,0.165613895153883,
-0.331484773207108));
#36905=CARTESIAN_POINT('Ctrl Pts',(-0.0955885941295399,0.156815213933875,
-0.320406892537285));
#36906=CARTESIAN_POINT('Ctrl Pts',(-0.155102372787945,0.0543511330211424,
-0.312913842321706));
#36907=CARTESIAN_POINT('Ctrl Pts',(-0.15579906137073,0.00152585119335764,
-0.309113418996068));
#36908=CARTESIAN_POINT('Ctrl Pts',(-0.155795396340587,2.73987766570313E-5,
-0.30900562256037));
#36909=CARTESIAN_POINT('Ctrl Pts',(-0.155793338978167,3.1743077477449E-5,
-0.36519437743963));
#36910=CARTESIAN_POINT('Ctrl Pts',(-0.155654352143183,-0.0495595560158264,
-0.361626978771191));
#36911=CARTESIAN_POINT('Ctrl Pts',(-0.103266255382889,-0.150735748184266,
-0.354366953212811));
#36912=CARTESIAN_POINT('Ctrl Pts',(0.0688325172648546,-0.170265295386756,
-0.343414300764493));
#36913=CARTESIAN_POINT('Ctrl Pts',(0.180268213518661,-0.0350935526860387,
-0.332336420094669));
#36914=CARTESIAN_POINT('Ctrl Pts',(0.127677660483707,0.132009852885846,
-0.321258539424848));
#36915=CARTESIAN_POINT('Ctrl Pts',(-0.0410869387683269,0.178997345541052,
-0.310180658755025));
#36916=CARTESIAN_POINT('Ctrl Pts',(-0.144124030240022,0.0881142143007613,
-0.301492604759952));
#36917=CARTESIAN_POINT('Ctrl Pts',(-0.155502498570681,0.0183419554515344,
-0.296497177654821));
#36918=CARTESIAN_POINT('Ctrl Pts',(-0.155384523600718,0.000108282706206955,
-0.29519437743963));
#36919=CARTESIAN_POINT('Origin',(0.,0.,-0.90400562256037));
#36920=CARTESIAN_POINT('',(-0.155346404813911,8.48772195699003E-5,-0.44900562256037));
#36921=CARTESIAN_POINT('',(-0.155471787680923,-0.000134750021813443,-0.43519437743963));
#36922=CARTESIAN_POINT('',(-0.15555,-8.39731161192283E-15,-0.90400562256037));
#36923=CARTESIAN_POINT('Ctrl Pts',(-0.155346404813911,8.48772195699028E-5,
-0.44900562256037));
#36924=CARTESIAN_POINT('Ctrl Pts',(-0.155189329744259,-0.0313878464499768,
-0.446758275008691));
#36925=CARTESIAN_POINT('Ctrl Pts',(-0.130644203207247,-0.114798780034182,
-0.440818300567071));
#36926=CARTESIAN_POINT('Ctrl Pts',(0.00527308248792088,-0.183576646798727,
-0.431185699235508));
#36927=CARTESIAN_POINT('Ctrl Pts',(0.15678546817529,-0.0956373756302127,
-0.420107818565687));
#36928=CARTESIAN_POINT('Ctrl Pts',(0.165638580847071,0.079322450689304,
-0.409029937895864));
#36929=CARTESIAN_POINT('Ctrl Pts',(0.023776963372566,0.182106690325406,
-0.397952057226042));
#36930=CARTESIAN_POINT('Ctrl Pts',(-0.123930728671449,0.125267447494704,
-0.38794395211421));
#36931=CARTESIAN_POINT('Ctrl Pts',(-0.155161147300025,0.0365271619785578,
-0.38162847389232));
#36932=CARTESIAN_POINT('Ctrl Pts',(-0.155465071756645,-0.000133606378324543,
-0.37900562256037));
#36933=CARTESIAN_POINT('Ctrl Pts',(-0.155471787680923,-0.000134750021813448,
-0.43519437743963));
#36934=CARTESIAN_POINT('Ctrl Pts',(-0.155595181194392,-0.0148422151223725,
-0.434142033667443));
#36935=CARTESIAN_POINT('Ctrl Pts',(-0.146947534876927,-0.0810153094256527,
-0.429397063005316));
#36936=CARTESIAN_POINT('Ctrl Pts',(-0.0530564558970885,-0.175821496790065,
-0.420959465453248));
#36937=CARTESIAN_POINT('Ctrl Pts',(0.11849103787925,-0.140314148210727,
-0.409881584783426));
#36938=CARTESIAN_POINT('Ctrl Pts',(0.182223403637476,0.0228652009081741,
-0.398803704113603));
#36939=CARTESIAN_POINT('Ctrl Pts',(0.0801504904255299,0.165239478122968,
-0.387725823443781));
#36940=CARTESIAN_POINT('Ctrl Pts',(-0.0948514437538827,0.15726216920691,
-0.376647942773958));
#36941=CARTESIAN_POINT('Ctrl Pts',(-0.154985099422088,0.0548408623920629,
-0.369137460772575));
#36942=CARTESIAN_POINT('Ctrl Pts',(-0.155798217904179,0.00177257183384377,
-0.365319605661132));
#36943=CARTESIAN_POINT('Ctrl Pts',(-0.155793338978167,3.1743077477449E-5,
-0.36519437743963));
#36944=CARTESIAN_POINT('Origin',(0.,0.,-0.90400562256037));
#36945=CARTESIAN_POINT('',(-0.155766976288708,6.54450248024079E-5,-0.51900562256037));
#36946=CARTESIAN_POINT('',(-0.155342420051734,8.16789539274873E-5,-0.50519437743963));
#36947=CARTESIAN_POINT('',(-0.15555,-8.39731161192283E-15,-0.90400562256037));
#36948=CARTESIAN_POINT('Ctrl Pts',(-0.155766976288708,6.54450248024148E-5,
-0.51900562256037));
#36949=CARTESIAN_POINT('Ctrl Pts',(-0.155513327568197,-0.0475667116816575,
-0.515580703015002));
#36950=CARTESIAN_POINT('Ctrl Pts',(-0.106744701507368,-0.147003556334546,
-0.508463156579693));
#36951=CARTESIAN_POINT('Ctrl Pts',(0.0622509536759654,-0.172780234487164,
-0.497652983254442));
#36952=CARTESIAN_POINT('Ctrl Pts',(0.178789470703585,-0.0419823273947417,
-0.48657510258462));
#36953=CARTESIAN_POINT('Ctrl Pts',(0.132647248167164,0.127015346310585,
-0.475497221914797));
#36954=CARTESIAN_POINT('Ctrl Pts',(-0.0341908539685392,0.180441614256847,
-0.464419341244976));
#36955=CARTESIAN_POINT('Ctrl Pts',(-0.142383830605297,0.0921530609529823,
-0.455588808126832));
#36956=CARTESIAN_POINT('Ctrl Pts',(-0.15544742049907,0.0203251276447392,
-0.450450901898631));
#36957=CARTESIAN_POINT('Ctrl Pts',(-0.155346404813911,8.48772195699028E-5,
-0.44900562256037));
#36958=CARTESIAN_POINT('Ctrl Pts',(-0.155342420051734,8.16789539274786E-5,
-0.50519437743963));
#36959=CARTESIAN_POINT('Ctrl Pts',(-0.155192669039577,-0.0311489244921932,
-0.502964461673755));
#36960=CARTESIAN_POINT('Ctrl Pts',(-0.130936243323583,-0.114309881666503,
-0.497041919017939));
#36961=CARTESIAN_POINT('Ctrl Pts',(0.00441131476189927,-0.183599364242272,
-0.487426749472182));
#36962=CARTESIAN_POINT('Ctrl Pts',(0.156334808549674,-0.0963722671792685,
-0.47634886880236));
#36963=CARTESIAN_POINT('Ctrl Pts',(0.166009085015979,0.0785440636680758,
-0.465270988132537));
#36964=CARTESIAN_POINT('Ctrl Pts',(0.0246315091798845,0.18199306305922,
-0.454193107462715));
#36965=CARTESIAN_POINT('Ctrl Pts',(-0.123599083728466,0.12574999846804,
-0.444167570565079));
#36966=CARTESIAN_POINT('Ctrl Pts',(-0.15516219891434,0.0367656173641079,
-0.437834660557384));
#36967=CARTESIAN_POINT('Ctrl Pts',(-0.155471787680923,-0.000134750021813448,
-0.43519437743963));
#36968=CARTESIAN_POINT('Origin',(0.,0.,-0.90400562256037));
#36969=CARTESIAN_POINT('',(-0.155529154618988,-0.000139780194698154,-0.58900562256037));
#36970=CARTESIAN_POINT('',(-0.155762681169959,6.92827665681687E-5,-0.57519437743963));
#36971=CARTESIAN_POINT('',(-0.15555,-8.39731161192283E-15,-0.90400562256037));
#36972=CARTESIAN_POINT('Ctrl Pts',(-0.155529154618988,-0.000139780194698135,
-0.58900562256037));
#36973=CARTESIAN_POINT('Ctrl Pts',(-0.155643250350289,-0.0128440365105712,
-0.588095757911254));
#36974=CARTESIAN_POINT('Ctrl Pts',(-0.148424039982469,-0.0769797460374569,
-0.583493266372197));
#36975=CARTESIAN_POINT('Ctrl Pts',(-0.0597614480239172,-0.173657013877139,
-0.575198147943198));
#36976=CARTESIAN_POINT('Ctrl Pts',(0.113021777413197,-0.144755894581878,
-0.564120267273377));
#36977=CARTESIAN_POINT('Ctrl Pts',(0.182966362384724,0.0158587828225596,
-0.553042386603554));
#36978=CARTESIAN_POINT('Ctrl Pts',(0.0864296486912397,0.162043532007437,
-0.541964505933732));
#36979=CARTESIAN_POINT('Ctrl Pts',(-0.0887494987382724,0.160784692096253,
-0.53088662526391));
#36980=CARTESIAN_POINT('Ctrl Pts',(-0.15398197464732,0.0588474973592622,
-0.523233664139455));
#36981=CARTESIAN_POINT('Ctrl Pts',(-0.155786802630472,0.00378859180802485,
-0.519273329904942));
#36982=CARTESIAN_POINT('Ctrl Pts',(-0.155766976288708,6.54450248024148E-5,
-0.51900562256037));
#36983=CARTESIAN_POINT('Ctrl Pts',(-0.155762681169959,6.9282766568167E-5,
-0.575194377439629));
#36984=CARTESIAN_POINT('Ctrl Pts',(-0.155497913037279,-0.0473238951863867,
-0.571786889680066));
#36985=CARTESIAN_POINT('Ctrl Pts',(-0.10716124014269,-0.146543711339655,
-0.564686775030562));
#36986=CARTESIAN_POINT('Ctrl Pts',(0.0614392328065822,-0.173070526112361,
-0.553894033491116));
#36987=CARTESIAN_POINT('Ctrl Pts',(0.178590424220399,-0.0428211002752123,
-0.542816152821293));
#36988=CARTESIAN_POINT('Ctrl Pts',(0.133241988508851,0.126391292087037,
-0.531738272151472));
#36989=CARTESIAN_POINT('Ctrl Pts',(-0.0333434816106114,0.180600106574017,
-0.520660391481649));
#36990=CARTESIAN_POINT('Ctrl Pts',(-0.142164078467833,0.092647109507526,
-0.511812426577702));
#36991=CARTESIAN_POINT('Ctrl Pts',(-0.155440649085617,0.0205673635573518,
-0.506657088563695));
#36992=CARTESIAN_POINT('Ctrl Pts',(-0.155342420051734,8.16789539274786E-5,
-0.50519437743963));
#36993=CARTESIAN_POINT('Origin',(0.,0.,-0.90400562256037));
#36994=CARTESIAN_POINT('',(-0.155316084506021,5.35377555358372E-5,-0.659005622560371));
#36995=CARTESIAN_POINT('',(-0.155536374284098,-0.000139852232319077,-0.64519437743963));
#36996=CARTESIAN_POINT('',(-0.15555,-8.39731161192283E-15,-0.90400562256037));
#36997=CARTESIAN_POINT('Ctrl Pts',(-0.155316084506021,5.3537755535819E-5,
-0.65900562256037));
#36998=CARTESIAN_POINT('Ctrl Pts',(-0.155225416432192,-0.0291940910521941,
-0.656918185917565));
#36999=CARTESIAN_POINT('Ctrl Pts',(-0.133259818681327,-0.110306616722607,
-0.65113812238482));
#37000=CARTESIAN_POINT('Ctrl Pts',(-0.00263426887515189,-0.183633273387178,
-0.641665431962132));
#37001=CARTESIAN_POINT('Ctrl Pts',(0.15252317418251,-0.102298032825963,
-0.630587551292311));
#37002=CARTESIAN_POINT('Ctrl Pts',(0.168899673978284,0.0721186645451872,
-0.619509670622488));
#37003=CARTESIAN_POINT('Ctrl Pts',(0.0315941379137935,0.180914318189617,
-0.608431789952666));
#37004=CARTESIAN_POINT('Ctrl Pts',(-0.120820410002026,0.129680488142133,
-0.598263773931959));
#37005=CARTESIAN_POINT('Ctrl Pts',(-0.155180200196799,0.038715366895471,
-0.591788384801195));
#37006=CARTESIAN_POINT('Ctrl Pts',(-0.155529154618988,-0.000139780194698135,
-0.58900562256037));
#37007=CARTESIAN_POINT('Ctrl Pts',(-0.155536374284098,-0.000139852232319075,
-0.64519437743963));
#37008=CARTESIAN_POINT('Ctrl Pts',(-0.155648810427832,-0.0125992364466732,
-0.644301944576318));
#37009=CARTESIAN_POINT('Ctrl Pts',(-0.148598384175115,-0.0764862520907471,
-0.639716884823065));
#37010=CARTESIAN_POINT('Ctrl Pts',(-0.0605759234386941,-0.17337454580915,
-0.631439198179872));
#37011=CARTESIAN_POINT('Ctrl Pts',(0.112341035698075,-0.145284827074641,
-0.62036131751005));
#37012=CARTESIAN_POINT('Ctrl Pts',(0.183038778318879,0.0149997688499129,
-0.609283436840227));
#37013=CARTESIAN_POINT('Ctrl Pts',(0.0871893223770248,0.161636031852426,
-0.598205556170405));
#37014=CARTESIAN_POINT('Ctrl Pts',(-0.0879937907449659,0.161199502407392,
-0.587127675500583));
#37015=CARTESIAN_POINT('Ctrl Pts',(-0.153853711608356,0.0593381461278729,
-0.579457282590324));
#37016=CARTESIAN_POINT('Ctrl Pts',(-0.155784837010399,0.00403515161213462,
-0.575479516570006));
#37017=CARTESIAN_POINT('Ctrl Pts',(-0.155762681169959,6.9282766568167E-5,
-0.575194377439629));
#37018=CARTESIAN_POINT('Origin',(0.,0.,-0.90400562256037));
#37019=CARTESIAN_POINT('',(-0.155718793124499,0.000108222005882066,-0.72900562256037));
#37020=CARTESIAN_POINT('',(-0.155313284670072,5.07842058497104E-5,-0.71519437743963));
#37021=CARTESIAN_POINT('',(-0.15555,-8.39731161192283E-15,-0.90400562256037));
#37022=CARTESIAN_POINT('Ctrl Pts',(-0.155718793124499,0.000108222005882058,
-0.72900562256037));
#37023=CARTESIAN_POINT('Ctrl Pts',(-0.155384204900034,-0.0453333351310797,
-0.725740613923876));
#37024=CARTESIAN_POINT('Ctrl Pts',(-0.110495670244879,-0.142777587024444,
-0.718782978397442));
#37025=CARTESIAN_POINT('Ctrl Pts',(0.0547571568913644,-0.175290438141162,
-0.708132715981067));
#37026=CARTESIAN_POINT('Ctrl Pts',(0.176815643105561,-0.0496447546162005,
-0.697054835311244));
#37027=CARTESIAN_POINT('Ctrl Pts',(0.137992423121185,0.121190070497784,
-0.685976954641421));
#37028=CARTESIAN_POINT('Ctrl Pts',(-0.0263918556098016,0.181744822170133,
-0.6748990739716));
#37029=CARTESIAN_POINT('Ctrl Pts',(-0.140311098627796,0.0966842315348642,
-0.665908629944582));
#37030=CARTESIAN_POINT('Ctrl Pts',(-0.155385806146838,0.0225442843254148,
-0.660610812807506));
#37031=CARTESIAN_POINT('Ctrl Pts',(-0.155316084506021,5.3537755535819E-5,
-0.65900562256037));
#37032=CARTESIAN_POINT('Ctrl Pts',(-0.155313284670072,5.07842058496948E-5,
-0.71519437743963));
#37033=CARTESIAN_POINT('Ctrl Pts',(-0.155229832237143,-0.0289541923389479,
-0.713124372582629));
#37034=CARTESIAN_POINT('Ctrl Pts',(-0.133537000198005,-0.109817572601608,
-0.707361740835688));
#37035=CARTESIAN_POINT('Ctrl Pts',(-0.00349579444440964,-0.183617766674194,
-0.697906482198806));
#37036=CARTESIAN_POINT('Ctrl Pts',(0.152041075972361,-0.103013424219718,
-0.686828601528983));
#37037=CARTESIAN_POINT('Ctrl Pts',(0.169236443271834,0.0713253547488333,
-0.675750720859162));
#37038=CARTESIAN_POINT('Ctrl Pts',(0.0324429392663866,0.18076385018324,
-0.664672840189339));
#37039=CARTESIAN_POINT('Ctrl Pts',(-0.120472031008651,0.130159640264286,
-0.654487392382829));
#37040=CARTESIAN_POINT('Ctrl Pts',(-0.155183582459629,0.0389540613681267,
-0.647994571466259));
#37041=CARTESIAN_POINT('Ctrl Pts',(-0.155536374284098,-0.000139852232319075,
-0.64519437743963));
#37042=CARTESIAN_POINT('Ctrl Pts',(-0.0685825729128701,0.139614588036676,
-0.797607408227207));
#37043=CARTESIAN_POINT('Ctrl Pts',(-0.114857746382803,0.116882934395126,
-0.793914781337266));
#37044=CARTESIAN_POINT('Ctrl Pts',(-0.182252520735991,0.0222053183358603,
-0.786529527557385));
#37045=CARTESIAN_POINT('Ctrl Pts',(-0.117832146183986,-0.141024052804591,
-0.775451646887562));
#37046=CARTESIAN_POINT('Ctrl Pts',(0.0539538561217182,-0.175492392417165,
-0.764373766217739));
#37047=CARTESIAN_POINT('Ctrl Pts',(0.176570107319903,-0.0505019485347378,
-0.753295885547919));
#37048=CARTESIAN_POINT('Ctrl Pts',(0.138565293653093,0.120555556476704,
-0.742218004878094));
#37049=CARTESIAN_POINT('Ctrl Pts',(-0.0255413571731973,0.181859045827175,
-0.731140124208274));
#37050=CARTESIAN_POINT('Ctrl Pts',(-0.166396812434887,0.0777204685530644,
-0.72006224353845));
#37051=CARTESIAN_POINT('Ctrl Pts',(-0.155853441635454,-0.0971526815038287,
-0.708984362868629));
#37052=CARTESIAN_POINT('Ctrl Pts',(-0.00349579444440964,-0.183617766674194,
-0.697906482198806));
#37053=CARTESIAN_POINT('Ctrl Pts',(0.152041075972361,-0.103013424219718,
-0.686828601528983));
#37054=CARTESIAN_POINT('Ctrl Pts',(0.169236443271834,0.0713253547488333,
-0.675750720859162));
#37055=CARTESIAN_POINT('Ctrl Pts',(0.0324429392663866,0.18076385018324,
-0.664672840189339));
#37056=CARTESIAN_POINT('Ctrl Pts',(-0.133870199391445,0.125725779248893,
-0.653594959519517));
#37057=CARTESIAN_POINT('Ctrl Pts',(-0.17837481560913,-0.0437106671942546,
-0.642517078849694));
#37058=CARTESIAN_POINT('Ctrl Pts',(-0.0605759234386941,-0.17337454580915,
-0.631439198179872));
#37059=CARTESIAN_POINT('Ctrl Pts',(0.112341035698075,-0.145284827074641,
-0.62036131751005));
#37060=CARTESIAN_POINT('Ctrl Pts',(0.183038778318879,0.0149997688499129,
-0.609283436840227));
#37061=CARTESIAN_POINT('Ctrl Pts',(0.0871893223770248,0.161636031852426,
-0.598205556170405));
#37062=CARTESIAN_POINT('Ctrl Pts',(-0.0879937907449659,0.161199502407392,
-0.587127675500583));
#37063=CARTESIAN_POINT('Ctrl Pts',(-0.18311125770977,0.0140873579667044,
-0.57604979483076));
#37064=CARTESIAN_POINT('Ctrl Pts',(-0.111615584950465,-0.145842885431028,
-0.564971914160939));
#37065=CARTESIAN_POINT('Ctrl Pts',(0.0614392328065822,-0.173070526112361,
-0.553894033491116));
#37066=CARTESIAN_POINT('Ctrl Pts',(0.178590424220399,-0.0428211002752123,
-0.542816152821293));
#37067=CARTESIAN_POINT('Ctrl Pts',(0.133241988508851,0.126391292087037,
-0.531738272151472));
#37068=CARTESIAN_POINT('Ctrl Pts',(-0.0333434816106114,0.180600106574017,
-0.520660391481649));
#37069=CARTESIAN_POINT('Ctrl Pts',(-0.169589680537707,0.0704806817533824,
-0.509582510811826));
#37070=CARTESIAN_POINT('Ctrl Pts',(-0.1515260392585,-0.103769194218193,
-0.498504630142005));
#37071=CARTESIAN_POINT('Ctrl Pts',(0.00441131476189927,-0.183599364242272,
-0.487426749472182));
#37072=CARTESIAN_POINT('Ctrl Pts',(0.156334808549674,-0.0963722671792685,
-0.47634886880236));
#37073=CARTESIAN_POINT('Ctrl Pts',(0.166009085015979,0.0785440636680758,
-0.465270988132537));
#37074=CARTESIAN_POINT('Ctrl Pts',(0.0246315091798845,0.18199306305922,
-0.454193107462715));
#37075=CARTESIAN_POINT('Ctrl Pts',(-0.139158304435279,0.119846370626905,
-0.443115226792893));
#37076=CARTESIAN_POINT('Ctrl Pts',(-0.17632782105536,-0.0513486686061268,
-0.43203734612307));
#37077=CARTESIAN_POINT('Ctrl Pts',(-0.0530564558970885,-0.175821496790065,
-0.420959465453248));
#37078=CARTESIAN_POINT('Ctrl Pts',(0.11849103787925,-0.140314148210727,
-0.409881584783426));
#37079=CARTESIAN_POINT('Ctrl Pts',(0.182223403637476,0.0228652009081741,
-0.398803704113603));
#37080=CARTESIAN_POINT('Ctrl Pts',(0.0801504904255299,0.165239478122968,
-0.387725823443781));
#37081=CARTESIAN_POINT('Ctrl Pts',(-0.0948514437538827,0.15726216920691,
-0.376647942773958));
#37082=CARTESIAN_POINT('Ctrl Pts',(-0.183547943074409,0.00619183647286117,
-0.365570062104137));
#37083=CARTESIAN_POINT('Ctrl Pts',(-0.105233963508669,-0.150512455198895,
-0.354492181434313));
#37084=CARTESIAN_POINT('Ctrl Pts',(0.0688325172648546,-0.170265295386756,
-0.343414300764493));
#37085=CARTESIAN_POINT('Ctrl Pts',(0.180268213518661,-0.0350935526860387,
-0.332336420094669));
#37086=CARTESIAN_POINT('Ctrl Pts',(0.127677660483707,0.132009852885846,
-0.321258539424848));
#37087=CARTESIAN_POINT('Ctrl Pts',(-0.0410869387683269,0.178997345541052,
-0.310180658755025));
#37088=CARTESIAN_POINT('Ctrl Pts',(-0.172466486424957,0.0631149530800074,
-0.299102778085203));
#37089=CARTESIAN_POINT('Ctrl Pts',(-0.146918585030578,-0.110195805809095,
-0.28802489741538));
#37090=CARTESIAN_POINT('Ctrl Pts',(0.0123107014066272,-0.183239277698152,
-0.276947016745558));
#37091=CARTESIAN_POINT('Ctrl Pts',(0.160338466762532,-0.0895531255371017,
-0.265869136075736));
#37092=CARTESIAN_POINT('Ctrl Pts',(0.162474081881463,0.0856175155489654,
-0.254791255405913));
#37093=CARTESIAN_POINT('Ctrl Pts',(0.0167743476807649,0.182884683876359,
-0.243713374736091));
#37094=CARTESIAN_POINT('Ctrl Pts',(-0.144188383635275,0.113744872672702,
-0.232635494066269));
#37095=CARTESIAN_POINT('Ctrl Pts',(-0.173953944439453,-0.0588915237406155,
-0.221557613396446));
#37096=CARTESIAN_POINT('Ctrl Pts',(-0.045438614211677,-0.177942460150977,
-0.210479732726624));
#37097=CARTESIAN_POINT('Ctrl Pts',(0.124421357682504,-0.135083346427328,
-0.199401852056802));
#37098=CARTESIAN_POINT('Ctrl Pts',(0.181070205071097,0.0306882431808897,
-0.18832397138698));
#37099=CARTESIAN_POINT('Ctrl Pts',(0.0729630546502829,0.168536589309041,
-0.177246090717157));
#37100=CARTESIAN_POINT('Ctrl Pts',(-0.1015332313447,0.153033259678028,-0.166168210047335));
#37101=CARTESIAN_POINT('Ctrl Pts',(-0.183644372729135,-0.0017151195528544,
-0.155090329377512));
#37102=CARTESIAN_POINT('Ctrl Pts',(-0.0986571866185378,-0.154903070922954,
-0.14401244870769));
#37103=CARTESIAN_POINT('Ctrl Pts',(0.0760980799328472,-0.16714423732766,
-0.132934568037868));
#37104=CARTESIAN_POINT('Ctrl Pts',(0.181612007146477,-0.027301260439323,
-0.121856687368045));
#37105=CARTESIAN_POINT('Ctrl Pts',(0.121876225192118,0.137384278886722,
-0.110778806698223));
#37106=CARTESIAN_POINT('Ctrl Pts',(-0.0487534599252984,0.177061585225392,
-0.0997009260284008));
#37107=CARTESIAN_POINT('Ctrl Pts',(-0.175025004118839,0.0556344023622128,
-0.0886230453585786));
#37108=CARTESIAN_POINT('Ctrl Pts',(-0.142035983272133,-0.116422291149579,
-0.0775451646887562));
#37109=CARTESIAN_POINT('Ctrl Pts',(0.0201819892413759,-0.182531533674816,
-0.0664672840189338));
#37110=CARTESIAN_POINT('Ctrl Pts',(0.164054917332699,-0.0825830908935778,
-0.0553894033491116));
#37111=CARTESIAN_POINT('Ctrl Pts',(0.158618708021993,0.0925610883157775,
-0.0443115226792891));
#37112=CARTESIAN_POINT('Ctrl Pts',(0.00892266599271826,0.183382072237952,
-0.0332336420094669));
#37113=CARTESIAN_POINT('Ctrl Pts',(-0.149021641743064,0.107539520344655,
-0.0221557613396447));
#37114=CARTESIAN_POINT('Ctrl Pts',(-0.171116143090106,-0.0665456463713913,
-0.0110778806698222));
#37115=CARTESIAN_POINT('Ctrl Pts',(-0.0824189364736414,-0.141637004936936,
-0.00369262688994078));
#37116=CARTESIAN_POINT('Ctrl Pts',(-0.0319621170202007,-0.152230829911641,
0.));
#37117=CARTESIAN_POINT('Ctrl Pts',(-0.0744392439309299,0.151537102412036,
-0.789938272151471));
#37118=CARTESIAN_POINT('Ctrl Pts',(-0.124666127810757,0.126864258590232,
-0.786245645261531));
#37119=CARTESIAN_POINT('Ctrl Pts',(-0.197816140046672,0.024101561635302,
-0.778860391481648));
#37120=CARTESIAN_POINT('Ctrl Pts',(-0.127894529180734,-0.153066929702187,
-0.767782510811827));
#37121=CARTESIAN_POINT('Ctrl Pts',(0.0585612946011998,-0.190478724438646,
-0.756704630142004));
#37122=CARTESIAN_POINT('Ctrl Pts',(0.191648471782987,-0.0548146082349622,
-0.745626749472183));
#37123=CARTESIAN_POINT('Ctrl Pts',(0.15039820258286,0.130850507565521,-0.734548868802359));
#37124=CARTESIAN_POINT('Ctrl Pts',(-0.0277224845349277,0.197389063991137,
-0.723470988132538));
#37125=CARTESIAN_POINT('Ctrl Pts',(-0.18060641915412,0.084357478457361,
-0.712393107462715));
#37126=CARTESIAN_POINT('Ctrl Pts',(-0.169162687642468,-0.105449122858007,
-0.701315226792893));
#37127=CARTESIAN_POINT('Ctrl Pts',(-0.00379432098166487,-0.199297972400041,
-0.690237346123071));
#37128=CARTESIAN_POINT('Ctrl Pts',(0.165024761555771,-0.111810349013795,
-0.679159465453248));
#37129=CARTESIAN_POINT('Ctrl Pts',(0.183688542841925,0.077416248109469,
-0.668081584783426));
#37130=CARTESIAN_POINT('Ctrl Pts',(0.0352134334906785,0.196200343121849,
-0.657003704113603));
#37131=CARTESIAN_POINT('Ctrl Pts',(-0.145302166488303,0.136462246200717,
-0.645925823443781));
#37132=CARTESIAN_POINT('Ctrl Pts',(-0.193607294773437,-0.0474433792647373,
-0.634847942773958));
#37133=CARTESIAN_POINT('Ctrl Pts',(-0.0657488593629036,-0.188180022398659,
-0.623770062104138));
#37134=CARTESIAN_POINT('Ctrl Pts',(0.121934500334457,-0.157691556655536,
-0.612692181434313));
#37135=CARTESIAN_POINT('Ctrl Pts',(0.198669540808984,0.016280687715591,
-0.601614300764494));
#37136=CARTESIAN_POINT('Ctrl Pts',(0.0946349336418375,0.175439087395807,
-0.590536420094668));
#37137=CARTESIAN_POINT('Ctrl Pts',(-0.0955081003157075,0.174965280122885,
-0.579458539424848));
#37138=CARTESIAN_POINT('Ctrl Pts',(-0.198748209643198,0.0152903606774588,
-0.568380658755025));
#37139=CARTESIAN_POINT('Ctrl Pts',(-0.121147099062276,-0.158297270911422,
-0.557302778085202));
#37140=CARTESIAN_POINT('Ctrl Pts',(0.0666858918172795,-0.187850040664119,
-0.546224897415381));
#37141=CARTESIAN_POINT('Ctrl Pts',(0.193841315477621,-0.0464778469718106,
-0.535147016745557));
#37142=CARTESIAN_POINT('Ctrl Pts',(0.144620308967606,0.137184591111291,
-0.524069136075737));
#37143=CARTESIAN_POINT('Ctrl Pts',(-0.0361908784651756,0.196022616478603,
-0.512991255405913));
#37144=CARTESIAN_POINT('Ctrl Pts',(-0.184071945124501,0.0764994434974575,
-0.501913374736091));
#37145=CARTESIAN_POINT('Ctrl Pts',(-0.164465742814594,-0.11263065867677,
-0.490835494066269));
#37146=CARTESIAN_POINT('Ctrl Pts',(0.00478802298703869,-0.199277998475755,
-0.479757613396446));
#37147=CARTESIAN_POINT('Ctrl Pts',(0.169685161320925,-0.104602064344369,
-0.468679732726624));
#37148=CARTESIAN_POINT('Ctrl Pts',(0.180185581400608,0.0852514052242152,
-0.457601852056802));
#37149=CARTESIAN_POINT('Ctrl Pts',(0.0267349392469986,0.197534525746265,
-0.446523971386979));
#37150=CARTESIAN_POINT('Ctrl Pts',(-0.151041854058649,0.13008076014685,
-0.435446090717158));
#37151=CARTESIAN_POINT('Ctrl Pts',(-0.191385495263131,-0.0557336347348181,
-0.424368210047334));
#37152=CARTESIAN_POINT('Ctrl Pts',(-0.0575872600704507,-0.190835932977966,
-0.413290329377513));
#37153=CARTESIAN_POINT('Ctrl Pts',(0.128609687529926,-0.152296402161649,
-0.40221244870769));
#37154=CARTESIAN_POINT('Ctrl Pts',(0.19778453646712,0.0248177954783882,
-0.391134568037868));
#37155=CARTESIAN_POINT('Ctrl Pts',(0.0869950142516475,0.179350253228936,
-0.380056687368046));
#37156=CARTESIAN_POINT('Ctrl Pts',(-0.102951368823189,0.170691714782599,
-0.368978806698223));
#37157=CARTESIAN_POINT('Ctrl Pts',(-0.199222186150622,0.00672059396443702,
-0.357900926028401));
#37158=CARTESIAN_POINT('Ctrl Pts',(-0.114220513269348,-0.163365602824901,
-0.346823045358578));
#37159=CARTESIAN_POINT('Ctrl Pts',(0.0747105325075507,-0.184805254716366,
-0.335745164688756));
#37160=CARTESIAN_POINT('Ctrl Pts',(0.195662381114758,-0.0380903984473996,
-0.324667284018934));
#37161=CARTESIAN_POINT('Ctrl Pts',(0.138580810103928,0.143282954005531,
-0.313589403349111));
#37162=CARTESIAN_POINT('Ctrl Pts',(-0.0445955951701644,0.194282986213528,
-0.30251152267929));
#37163=CARTESIAN_POINT('Ctrl Pts',(-0.187194418459746,0.0685047117433281,
-0.291433642009467));
#37164=CARTESIAN_POINT('Ctrl Pts',(-0.159464830853934,-0.119606076593391,
-0.280355761339645));
#37165=CARTESIAN_POINT('Ctrl Pts',(0.0133619849190106,-0.198887162014602,
-0.269277880669822));
#37166=CARTESIAN_POINT('Ctrl Pts',(0.174030715558174,-0.0972005959167307,
-0.2582));
#37167=CARTESIAN_POINT('Ctrl Pts',(0.176348703467184,0.0929289009440708,
-0.247122119330178));
#37168=CARTESIAN_POINT('Ctrl Pts',(0.0182068083152422,0.198502287331782,
-0.236044238660356));
#37169=CARTESIAN_POINT('Ctrl Pts',(-0.156501481434194,0.12345821924081,
-0.224966357990533));
#37170=CARTESIAN_POINT('Ctrl Pts',(-0.18880889930051,-0.063920618824861,
-0.213888477320711));
#37171=CARTESIAN_POINT('Ctrl Pts',(-0.049318885884956,-0.19313801792879,
-0.202810596650889));
#37172=CARTESIAN_POINT('Ctrl Pts',(0.135046432371559,-0.146618911315637,
-0.191732715981066));
#37173=CARTESIAN_POINT('Ctrl Pts',(0.196532859463218,0.0333088935414555,
-0.180654835311244));
#37174=CARTESIAN_POINT('Ctrl Pts',(0.0791938008793927,0.182928924215213,
-0.169576954641422));
#37175=CARTESIAN_POINT('Ctrl Pts',(-0.110203753725683,0.166101673688893,
-0.158499073971599));
#37176=CARTESIAN_POINT('Ctrl Pts',(-0.199326850503175,-0.00186158374267733,
-0.147421193301777));
#37177=CARTESIAN_POINT('Ctrl Pts',(-0.107082106551569,-0.16813115916099,
-0.136343312631954));
#37178=CARTESIAN_POINT('Ctrl Pts',(0.0825965444894176,-0.181417671073524,
-0.125265431962133));
#37179=CARTESIAN_POINT('Ctrl Pts',(0.197120929218237,-0.0296326763366925,
-0.11418755129231));
#37180=CARTESIAN_POINT('Ctrl Pts',(0.132283955983731,0.149116333989338,
-0.103109670622488));
#37181=CARTESIAN_POINT('Ctrl Pts',(-0.0529168058548446,0.192181919889984,
-0.0920317899526653));
#37182=CARTESIAN_POINT('Ctrl Pts',(-0.189971423092665,0.060385352612153,
-0.080953909282843));
#37183=CARTESIAN_POINT('Ctrl Pts',(-0.154165274889822,-0.126364278296928,
-0.0698760286130208));
#37184=CARTESIAN_POINT('Ctrl Pts',(0.0219054485176395,-0.198118979548471,
-0.0587981479431983));
#37185=CARTESIAN_POINT('Ctrl Pts',(0.178064535795589,-0.0896353488430248,
-0.047720267273376));
#37186=CARTESIAN_POINT('Ctrl Pts',(0.172164096460172,0.100465426405102,
-0.0366423866035536));
#37187=CARTESIAN_POINT('Ctrl Pts',(0.0096846251479957,0.199042150623642,
-0.0255645059337314));
#37188=CARTESIAN_POINT('Ctrl Pts',(-0.161747480001847,0.116722955222475,
-0.0144866252639091));
#37189=CARTESIAN_POINT('Ctrl Pts',(-0.185728761331059,-0.0722283721999558,
-0.00340874459408669));
#37190=CARTESIAN_POINT('Ctrl Pts',(-0.0894571763075103,-0.153732225437818,
0.00397650918579475));
#37191=CARTESIAN_POINT('Ctrl Pts',(-0.0346915509926754,-0.165230719704803,
0.00766913607573553));
#37192=CARTESIAN_POINT('Ctrl Pts',(-0.0802959149489896,0.163459616787396,
-0.782269136075736));
#37193=CARTESIAN_POINT('Ctrl Pts',(-0.13447450923871,0.136845582785338,
-0.778576509185795));
#37194=CARTESIAN_POINT('Ctrl Pts',(-0.213379759357353,0.0259978049347435,
-0.771191255405914));
#37195=CARTESIAN_POINT('Ctrl Pts',(-0.137956912177481,-0.165109806599782,
-0.760113374736091));
#37196=CARTESIAN_POINT('Ctrl Pts',(0.0631687330806816,-0.205465056460127,
-0.749035494066269));
#37197=CARTESIAN_POINT('Ctrl Pts',(0.20672683624607,-0.0591272679351864,
-0.737957613396446));
#37198=CARTESIAN_POINT('Ctrl Pts',(0.162231111512628,0.141145458654337,
-0.726879732726624));
#37199=CARTESIAN_POINT('Ctrl Pts',(-0.0299036118966582,0.212919082155099,
-0.715801852056802));
#37200=CARTESIAN_POINT('Ctrl Pts',(-0.194816025873353,0.0909944883616574,
-0.704723971386979));
#37201=CARTESIAN_POINT('Ctrl Pts',(-0.182471933649482,-0.113745564212185,
-0.693646090717158));
#37202=CARTESIAN_POINT('Ctrl Pts',(-0.00409284751891995,-0.214978178125889,
-0.682568210047334));
#37203=CARTESIAN_POINT('Ctrl Pts',(0.178008447139181,-0.120607273807872,
-0.671490329377513));
#37204=CARTESIAN_POINT('Ctrl Pts',(0.198140642412015,0.0835071414701047,
-0.66041244870769));
#37205=CARTESIAN_POINT('Ctrl Pts',(0.0379839277149706,0.211636836060458,
-0.649334568037868));
#37206=CARTESIAN_POINT('Ctrl Pts',(-0.156734133585161,0.147198713152541,
-0.638256687368046));
#37207=CARTESIAN_POINT('Ctrl Pts',(-0.208839773937744,-0.0511760913352197,
-0.627178806698223));
#37208=CARTESIAN_POINT('Ctrl Pts',(-0.0709217952871131,-0.202985498988168,
-0.616100926028401));
#37209=CARTESIAN_POINT('Ctrl Pts',(0.13152796497084,-0.170098286236431,
-0.605023045358579));
#37210=CARTESIAN_POINT('Ctrl Pts',(0.214300303299088,0.0175616065812689,
-0.593945164688756));
#37211=CARTESIAN_POINT('Ctrl Pts',(0.10208054490665,0.189242142939189,-0.582867284018934));
#37212=CARTESIAN_POINT('Ctrl Pts',(-0.103022409886449,0.188731057838378,
-0.571789403349112));
#37213=CARTESIAN_POINT('Ctrl Pts',(-0.214385161576627,0.0164933633882133,
-0.560711522679289));
#37214=CARTESIAN_POINT('Ctrl Pts',(-0.130678613174086,-0.170751656391817,
-0.549633642009467));
#37215=CARTESIAN_POINT('Ctrl Pts',(0.0719325508279769,-0.202629555215876,
-0.538555761339645));
#37216=CARTESIAN_POINT('Ctrl Pts',(0.209092206734844,-0.050134593668409,
-0.527477880669822));
#37217=CARTESIAN_POINT('Ctrl Pts',(0.155998629426361,0.147977890135545,
-0.5164));
#37218=CARTESIAN_POINT('Ctrl Pts',(-0.0390382753197402,0.211445126383187,
-0.505322119330178));
#37219=CARTESIAN_POINT('Ctrl Pts',(-0.198554209711295,0.0825182052415327,
-0.494244238660355));
#37220=CARTESIAN_POINT('Ctrl Pts',(-0.177405446370688,-0.121492123135346,
-0.483166357990533));
#37221=CARTESIAN_POINT('Ctrl Pts',(0.00516473121217803,-0.214956632709237,
-0.472088477320711));
#37222=CARTESIAN_POINT('Ctrl Pts',(0.183035514092176,-0.11283186150947,
-0.461010596650888));
#37223=CARTESIAN_POINT('Ctrl Pts',(0.194362077785237,0.0919587467803548,
-0.449932715981067));
#37224=CARTESIAN_POINT('Ctrl Pts',(0.0288383693141127,0.213075988433311,
-0.438854835311244));
#37225=CARTESIAN_POINT('Ctrl Pts',(-0.162925403682019,0.140315149666796,
-0.427776954641422));
#37226=CARTESIAN_POINT('Ctrl Pts',(-0.206443169470902,-0.0601186008635093,
-0.416699073971599));
#37227=CARTESIAN_POINT('Ctrl Pts',(-0.0621180642438127,-0.205850369165867,
-0.405621193301777));
#37228=CARTESIAN_POINT('Ctrl Pts',(0.138728337180602,-0.164278656112571,
-0.394543312631955));
#37229=CARTESIAN_POINT('Ctrl Pts',(0.213345669296764,0.0267703900486021,
-0.383465431962132));
#37230=CARTESIAN_POINT('Ctrl Pts',(0.093839538077765,0.193461028334904,
-0.37238755129231));
#37231=CARTESIAN_POINT('Ctrl Pts',(-0.111051293892496,0.184121260358289,
-0.361309670622487));
#37232=CARTESIAN_POINT('Ctrl Pts',(-0.214896429226836,0.00724935145601278,
-0.350231789952666));
#37233=CARTESIAN_POINT('Ctrl Pts',(-0.123207063030027,-0.176218750450907,
-0.339153909282843));
#37234=CARTESIAN_POINT('Ctrl Pts',(0.0805885477502469,-0.199345214045976,
-0.328076028613021));
#37235=CARTESIAN_POINT('Ctrl Pts',(0.211056548710855,-0.0410872442087603,
-0.316998147943199));
#37236=CARTESIAN_POINT('Ctrl Pts',(0.149483959724149,0.154556055125215,
-0.305920267273376));
#37237=CARTESIAN_POINT('Ctrl Pts',(-0.048104251572002,0.209568626886004,
-0.294842386603554));
#37238=CARTESIAN_POINT('Ctrl Pts',(-0.201922350494536,0.073894470406649,
-0.283764505933731));
#37239=CARTESIAN_POINT('Ctrl Pts',(-0.172011076677289,-0.129016347377688,
-0.272686625263909));
#37240=CARTESIAN_POINT('Ctrl Pts',(0.014413268431394,-0.214535046331052,
-0.261608744594087));
#37241=CARTESIAN_POINT('Ctrl Pts',(0.187722964353817,-0.10484806629636,
-0.250530863924265));
#37242=CARTESIAN_POINT('Ctrl Pts',(0.190223325052905,0.100240286339176,
-0.239452983254442));
#37243=CARTESIAN_POINT('Ctrl Pts',(0.0196392689497196,0.214119890787204,
-0.22837510258462));
#37244=CARTESIAN_POINT('Ctrl Pts',(-0.168814579233112,0.133171565808918,
-0.217297221914798));
#37245=CARTESIAN_POINT('Ctrl Pts',(-0.203663854161568,-0.0689497139091067,
-0.206219341244975));
#37246=CARTESIAN_POINT('Ctrl Pts',(-0.053199157558235,-0.208333575706603,
-0.195141460575153));
#37247=CARTESIAN_POINT('Ctrl Pts',(0.145671507060614,-0.158154476203945,
-0.184063579905331));
#37248=CARTESIAN_POINT('Ctrl Pts',(0.211995513855339,0.0359295439020216,
-0.172985699235508));
#37249=CARTESIAN_POINT('Ctrl Pts',(0.0854245471085026,0.197321259121385,
-0.161907818565686));
#37250=CARTESIAN_POINT('Ctrl Pts',(-0.118874276106667,0.179170087699757,
-0.150829937895864));
#37251=CARTESIAN_POINT('Ctrl Pts',(-0.215009328277216,-0.00200804793250031,
-0.139752057226041));
#37252=CARTESIAN_POINT('Ctrl Pts',(-0.1155070264846,-0.181359247399026,
-0.128674176556219));
#37253=CARTESIAN_POINT('Ctrl Pts',(0.0890950090459882,-0.195691104819388,
-0.117596295886397));
#37254=CARTESIAN_POINT('Ctrl Pts',(0.212629851289998,-0.0319640922340619,
-0.106518415216574));
#37255=CARTESIAN_POINT('Ctrl Pts',(0.142691686775344,0.160848389091954,
-0.0954405345467522));
#37256=CARTESIAN_POINT('Ctrl Pts',(-0.0570801517843907,0.207302254554576,
-0.0843626538769298));
#37257=CARTESIAN_POINT('Ctrl Pts',(-0.20491784206649,0.0651363028620932,
-0.0732847732071075));
#37258=CARTESIAN_POINT('Ctrl Pts',(-0.166294566507511,-0.136306265444277,
-0.0622068925372852));
#37259=CARTESIAN_POINT('Ctrl Pts',(0.0236289077939032,-0.213706425422127,
-0.0511290118674628));
#37260=CARTESIAN_POINT('Ctrl Pts',(0.19207415425848,-0.0966876067924717,
-0.0400511311976405));
#37261=CARTESIAN_POINT('Ctrl Pts',(0.185709484898353,0.108369764494427,
-0.0289732505278181));
#37262=CARTESIAN_POINT('Ctrl Pts',(0.0104465843032729,0.214702229009333,
-0.0178953698579959));
#37263=CARTESIAN_POINT('Ctrl Pts',(-0.174473318260629,0.125906390100295,
-0.00681748918817361));
#37264=CARTESIAN_POINT('Ctrl Pts',(-0.200341379572013,-0.07791109802852,
0.00426039148164884));
#37265=CARTESIAN_POINT('Ctrl Pts',(-0.0964954161413792,-0.165827445938701,
0.0116456452615303));
#37266=CARTESIAN_POINT('Ctrl Pts',(-0.0374209849651502,-0.178230609497964,
0.0153382721514711));
#37267=CARTESIAN_POINT('Ctrl Pts',(-0.0861525859670493,0.175382131162756,
-0.7746));
#37268=CARTESIAN_POINT('Ctrl Pts',(-0.144282890666663,0.146826906980443,
-0.77090737311006));
#37269=CARTESIAN_POINT('Ctrl Pts',(-0.228943378668034,0.0278940482341852,
-0.763522119330178));
#37270=CARTESIAN_POINT('Ctrl Pts',(-0.148019295174229,-0.177152683497377,
-0.752444238660355));
#37271=CARTESIAN_POINT('Ctrl Pts',(0.067776171560163,-0.220451388481608,
-0.741366357990533));
#37272=CARTESIAN_POINT('Ctrl Pts',(0.221805200709154,-0.0634399276354107,
-0.730288477320711));
#37273=CARTESIAN_POINT('Ctrl Pts',(0.174064020442395,0.151440409743154,
-0.719210596650888));
#37274=CARTESIAN_POINT('Ctrl Pts',(-0.0320847392583885,0.228449100319062,
-0.708132715981067));
#37275=CARTESIAN_POINT('Ctrl Pts',(-0.209025632592586,0.097631498265954,
-0.697054835311244));
#37276=CARTESIAN_POINT('Ctrl Pts',(-0.195781179656496,-0.122042005566363,
-0.685976954641422));
#37277=CARTESIAN_POINT('Ctrl Pts',(-0.00439137405617511,-0.230658383851736,
-0.674899073971599));
#37278=CARTESIAN_POINT('Ctrl Pts',(0.190992132722591,-0.129404198601949,
-0.663821193301777));
#37279=CARTESIAN_POINT('Ctrl Pts',(0.212592741982105,0.0895980348307404,
-0.652743312631955));
#37280=CARTESIAN_POINT('Ctrl Pts',(0.0407544219392627,0.227073328999068,
-0.641665431962132));
#37281=CARTESIAN_POINT('Ctrl Pts',(-0.168166100682019,0.157935180104365,
-0.630587551292311));
#37282=CARTESIAN_POINT('Ctrl Pts',(-0.224072253102051,-0.0549088034057021,
-0.619509670622487));
#37283=CARTESIAN_POINT('Ctrl Pts',(-0.0760947312113224,-0.217790975577677,
-0.608431789952666));
#37284=CARTESIAN_POINT('Ctrl Pts',(0.141121429607223,-0.182505015817326,
-0.597353909282842));
#37285=CARTESIAN_POINT('Ctrl Pts',(0.229931065789193,0.0188425254469469,
-0.586276028613023));
#37286=CARTESIAN_POINT('Ctrl Pts',(0.109526156171463,0.20304519848257,-0.575198147943197));
#37287=CARTESIAN_POINT('Ctrl Pts',(-0.110536719457191,0.202496835553871,
-0.564120267273377));
#37288=CARTESIAN_POINT('Ctrl Pts',(-0.230022113510055,0.0176963660989677,
-0.553042386603553));
#37289=CARTESIAN_POINT('Ctrl Pts',(-0.140210127285897,-0.183206041872212,
-0.541964505933732));
#37290=CARTESIAN_POINT('Ctrl Pts',(0.0771792098386744,-0.217409069767634,
-0.530886625263909));
#37291=CARTESIAN_POINT('Ctrl Pts',(0.224343097992066,-0.0537913403650071,
-0.519808744594087));
#37292=CARTESIAN_POINT('Ctrl Pts',(0.167376949885116,0.158771189159799,
-0.508730863924265));
#37293=CARTESIAN_POINT('Ctrl Pts',(-0.0418856721743048,0.226867636287773,
-0.497652983254443));
#37294=CARTESIAN_POINT('Ctrl Pts',(-0.213036474298089,0.0885369669856078,
-0.486575102584619));
#37295=CARTESIAN_POINT('Ctrl Pts',(-0.190345149926783,-0.130353587593923,
-0.475497221914798));
#37296=CARTESIAN_POINT('Ctrl Pts',(0.00554143943731765,-0.230635266942719,
-0.464419341244975));
#37297=CARTESIAN_POINT('Ctrl Pts',(0.196385866863427,-0.121061658674571,
-0.453341460575153));
#37298=CARTESIAN_POINT('Ctrl Pts',(0.208538574169865,0.0986660883364943,
-0.442263579905331));
#37299=CARTESIAN_POINT('Ctrl Pts',(0.0309417993812268,0.228617451120356,
-0.431185699235508));
#37300=CARTESIAN_POINT('Ctrl Pts',(-0.174808953305389,0.150549539186741,
-0.420107818565687));
#37301=CARTESIAN_POINT('Ctrl Pts',(-0.221500843678673,-0.0645035669922008,
-0.409029937895863));
#37302=CARTESIAN_POINT('Ctrl Pts',(-0.0666488684171745,-0.220864805353768,
-0.397952057226042));
#37303=CARTESIAN_POINT('Ctrl Pts',(0.148846986831278,-0.176260910063493,
-0.386874176556219));
#37304=CARTESIAN_POINT('Ctrl Pts',(0.228906802126409,0.028722984618816,
-0.375796295886397));
#37305=CARTESIAN_POINT('Ctrl Pts',(0.100684061903882,0.207571803440873,
-0.364718415216575));
#37306=CARTESIAN_POINT('Ctrl Pts',(-0.119151218961802,0.197550805933978,
-0.353640534546752));
#37307=CARTESIAN_POINT('Ctrl Pts',(-0.23057067230305,0.00777810894758914,
-0.34256265387693));
#37308=CARTESIAN_POINT('Ctrl Pts',(-0.132193612790705,-0.189071898076914,
-0.331484773207107));
#37309=CARTESIAN_POINT('Ctrl Pts',(0.0864665629929426,-0.213885173375585,
-0.320406892537285));
#37310=CARTESIAN_POINT('Ctrl Pts',(0.226450716306952,-0.0440840899701212,
-0.309329011867463));
#37311=CARTESIAN_POINT('Ctrl Pts',(0.16038710934437,0.1658291562449,-0.298251131197641));
#37312=CARTESIAN_POINT('Ctrl Pts',(-0.0516129079738391,0.224854267558481,
-0.287173250527818));
#37313=CARTESIAN_POINT('Ctrl Pts',(-0.216650282529325,0.0792842290699699,
-0.276095369857996));
#37314=CARTESIAN_POINT('Ctrl Pts',(-0.184557322500644,-0.138426618161985,
-0.265017489188174));
#37315=CARTESIAN_POINT('Ctrl Pts',(0.0154645519437773,-0.230182930647502,
-0.253939608518351));
#37316=CARTESIAN_POINT('Ctrl Pts',(0.20141521314946,-0.112495536675989,
-0.242861727848529));
#37317=CARTESIAN_POINT('Ctrl Pts',(0.204097946638625,0.107551671734282,
-0.231783847178707));
#37318=CARTESIAN_POINT('Ctrl Pts',(0.021071729584197,0.229737494242626,
-0.220705966508885));
#37319=CARTESIAN_POINT('Ctrl Pts',(-0.181127677032031,0.142884912377025,
-0.209628085839062));
#37320=CARTESIAN_POINT('Ctrl Pts',(-0.218518809022625,-0.0739788089933519,
-0.19855020516924));
#37321=CARTESIAN_POINT('Ctrl Pts',(-0.0570794292315143,-0.223529133484416,
-0.187472324499417));
#37322=CARTESIAN_POINT('Ctrl Pts',(0.156296581749669,-0.169690041092254,
-0.176394443829595));
#37323=CARTESIAN_POINT('Ctrl Pts',(0.22745816824746,0.0385501942625873,
-0.165316563159773));
#37324=CARTESIAN_POINT('Ctrl Pts',(0.0916552933376127,0.211713594027557,
-0.154238682489951));
#37325=CARTESIAN_POINT('Ctrl Pts',(-0.127544798487651,0.19223850171062,
-0.143160801820128));
#37326=CARTESIAN_POINT('Ctrl Pts',(-0.230691806051256,-0.00215451212232307,
-0.132082921150306));
#37327=CARTESIAN_POINT('Ctrl Pts',(-0.123931946417632,-0.194587335637062,
-0.121005040480483));
#37328=CARTESIAN_POINT('Ctrl Pts',(0.0955934736025586,-0.209964538565252,
-0.109927159810661));
#37329=CARTESIAN_POINT('Ctrl Pts',(0.228138773361758,-0.0342955081314312,
-0.0988492791408387));
#37330=CARTESIAN_POINT('Ctrl Pts',(0.153099417566957,0.172580444194569,
-0.0877713984710167));
#37331=CARTESIAN_POINT('Ctrl Pts',(-0.0612434977139372,0.222422589219168,
-0.0766935178011943));
#37332=CARTESIAN_POINT('Ctrl Pts',(-0.219864261040315,0.0698872531120333,
-0.065615637131372));
#37333=CARTESIAN_POINT('Ctrl Pts',(-0.178423858125201,-0.146248252591626,
-0.0545377564615497));
#37334=CARTESIAN_POINT('Ctrl Pts',(0.025352367070167,-0.229293871295783,
-0.0434598757917272));
#37335=CARTESIAN_POINT('Ctrl Pts',(0.20608377272137,-0.103739864741919,
-0.032381995121905));
#37336=CARTESIAN_POINT('Ctrl Pts',(0.199254873336532,0.116274102583752,
-0.0213041144520825));
#37337=CARTESIAN_POINT('Ctrl Pts',(0.0112085434585504,0.230362307395023,
-0.0102262337822604));
#37338=CARTESIAN_POINT('Ctrl Pts',(-0.187199156519412,0.135089824978115,
0.000851646887561937));
#37339=CARTESIAN_POINT('Ctrl Pts',(-0.214953997812966,-0.0835938238570844,
0.0119295275573844));
#37340=CARTESIAN_POINT('Ctrl Pts',(-0.103533655975248,-0.177922666439583,
0.0193147813372658));
#37341=CARTESIAN_POINT('Ctrl Pts',(-0.0401504189376249,-0.191230499291126,
0.0230074082272066));
#37342=CARTESIAN_POINT('',(-0.14957294282862,0.126218275177078,2.60208521396521E-16));
#37343=CARTESIAN_POINT('Ctrl Pts',(-0.149572942828615,0.126218275177084,
-1.90819582357449E-16));
#37344=CARTESIAN_POINT('Ctrl Pts',(-0.152409355584855,0.12213839882076,
-1.87889127479728E-16));
#37345=CARTESIAN_POINT('Ctrl Pts',(-0.155074825311664,0.117949841983875,
-2.1390244607528E-16));
#37346=CARTESIAN_POINT('Ctrl Pts',(-0.157558539584755,0.113656763614523,
-2.04697370165263E-16));
#37347=CARTESIAN_POINT('Ctrl Pts',(-0.162058150554841,0.105879225459084,
-1.88083489625304E-16));
#37348=CARTESIAN_POINT('Ctrl Pts',(-0.165961946681547,0.0977586786429782,
-1.12184872298018E-16));
#37349=CARTESIAN_POINT('Ctrl Pts',(-0.16926637762541,0.0893686620215524,
-8.32667268468867E-17));
#37350=CARTESIAN_POINT('Ctrl Pts',(-0.171514642330858,0.0836602727198771,
-6.35914342263728E-17));
#37351=CARTESIAN_POINT('Ctrl Pts',(-0.173486025552789,0.0778223415514922,
-5.15165993817366E-17));
#37352=CARTESIAN_POINT('Ctrl Pts',(-0.175169499051515,0.0719067612362681,
-5.55111512312578E-17));
#37353=CARTESIAN_POINT('Ctrl Pts',(-0.177114241837621,0.0650731032354923,
-6.01256437664607E-17));
#37354=CARTESIAN_POINT('Ctrl Pts',(-0.178678026440626,0.058129532159444,
-1.80244693759025E-17));
#37355=CARTESIAN_POINT('Ctrl Pts',(-0.179858327438416,0.0511127445516475,
-7.28583859910259E-17));
#37356=CARTESIAN_POINT('Ctrl Pts',(-0.18088836409873,0.0449892654669132,
-1.2071138657974E-16));
#37357=CARTESIAN_POINT('Ctrl Pts',(-0.181626262306867,0.0388099715919878,
1.20909457254854E-16));
#37358=CARTESIAN_POINT('Ctrl Pts',(-0.182067201079106,0.0325999030412639,
1.59594559789866E-16));
#37359=CARTESIAN_POINT('Ctrl Pts',(-0.182359376173048,0.028484983972151,
1.85228103898386E-16));
#37360=CARTESIAN_POINT('Ctrl Pts',(-0.182520385982331,0.0243657260406017,
2.37793219281459E-16));
#37361=CARTESIAN_POINT('Ctrl Pts',(-0.182550077425778,0.0202529927329005,
2.18575157973078E-16));
#37362=CARTESIAN_POINT('Ctrl Pts',(-0.182638158679569,0.00805234957811116,
1.61563752027702E-16));
#37363=CARTESIAN_POINT('Ctrl Pts',(-0.181574880217677,-0.00410296492725809,
-4.2435135068192E-18));
#37364=CARTESIAN_POINT('Ctrl Pts',(-0.17933098841831,-0.01602004498147,
-3.29597460435593E-17));
#37365=CARTESIAN_POINT('Ctrl Pts',(-0.178221946841473,-0.0219100514685647,
-4.71527190836742E-17));
#37366=CARTESIAN_POINT('Ctrl Pts',(-0.176823766898375,-0.0277415985898121,
-1.23108892831518E-16));
#37367=CARTESIAN_POINT('Ctrl Pts',(-0.175128724846193,-0.0334888034719142,
-1.196959198424E-16));
#37368=CARTESIAN_POINT('Ctrl Pts',(-0.174065414734053,-0.0370940597897774,
-1.17554941282537E-16));
#37369=CARTESIAN_POINT('Ctrl Pts',(-0.172884634981322,-0.0406668331426877,
4.85499834843578E-16));
#37370=CARTESIAN_POINT('Ctrl Pts',(-0.171590404833548,-0.0441852584481628,
4.28476698566271E-16));
#37371=CARTESIAN_POINT('Ctrl Pts',(-0.169183900073534,-0.050727454409171,
3.22447296362707E-16));
#37372=CARTESIAN_POINT('Ctrl Pts',(-0.166382027562676,-0.0570950810552904,
-3.16274383796401E-17));
#37373=CARTESIAN_POINT('Ctrl Pts',(-0.163177510429029,-0.0632495561099533,
-3.46944695195361E-18));
#37374=CARTESIAN_POINT('Ctrl Pts',(-0.159378089464225,-0.0705465810827711,
2.98008237155791E-17));
#37375=CARTESIAN_POINT('Ctrl Pts',(-0.155012614776842,-0.0775443065037668,
1.01748044056608E-16));
#37376=CARTESIAN_POINT('Ctrl Pts',(-0.150134094058049,-0.0842019941615851,
1.47451495458029E-16));
#37377=CARTESIAN_POINT('Ctrl Pts',(-0.147447444266624,-0.0878684488490376,
1.72620839866475E-16));
#37378=CARTESIAN_POINT('Ctrl Pts',(-0.144605056887674,-0.0914316066797669,
4.6437475298905E-17));
#37379=CARTESIAN_POINT('Ctrl Pts',(-0.141615068278682,-0.094883245817762,
-1.21430643318376E-17));
#37380=CARTESIAN_POINT('Ctrl Pts',(-0.139243928227529,-0.0976204869489193,
-5.85989816951453E-17));
#37381=CARTESIAN_POINT('Ctrl Pts',(-0.136785305582189,-0.100281264847667,
-5.84262065888997E-17));
#37382=CARTESIAN_POINT('Ctrl Pts',(-0.134247412155013,-0.102859257524588,
-4.5102810375397E-17));
#37383=CARTESIAN_POINT('Ctrl Pts',(-0.127464722402785,-0.109749115200969,
-9.49514379865841E-18));
#37384=CARTESIAN_POINT('Ctrl Pts',(-0.120109608121736,-0.116057478078322,
-2.73862375609035E-17));
#37385=CARTESIAN_POINT('Ctrl Pts',(-0.112270412127471,-0.121716646311139,
6.07153216591882E-18));
#37386=CARTESIAN_POINT('Ctrl Pts',(-0.107173860027412,-0.125395881498351,
2.78236693352516E-17));
#37387=CARTESIAN_POINT('Ctrl Pts',(-0.101872390808594,-0.128800281258816,
1.78627078510015E-16));
#37388=CARTESIAN_POINT('Ctrl Pts',(-0.0963888361066501,-0.131905437921845,
1.97758476261356E-16));
#37389=CARTESIAN_POINT('Ctrl Pts',(-0.092445112883218,-0.134138638666618,
2.11517605459416E-16));
#37390=CARTESIAN_POINT('Ctrl Pts',(-0.0884032420310201,-0.13621834887122,
-2.35626616501682E-16));
#37391=CARTESIAN_POINT('Ctrl Pts',(-0.0842970527965122,-0.138123431873126,
-2.03396327558281E-16));
#37392=CARTESIAN_POINT('Ctrl Pts',(-0.0745227262503713,-0.142658269966226,
-1.26675711235531E-16));
#37393=CARTESIAN_POINT('Ctrl Pts',(-0.0643598268954344,-0.146223024533765,
-1.39475126112393E-16));
#37394=CARTESIAN_POINT('Ctrl Pts',(-0.0539300424733775,-0.148702066835777,
-1.03432887255117E-16));
#37395=CARTESIAN_POINT('Ctrl Pts',(-0.0467211978956824,-0.150415528009428,
-7.85212603565983E-17));
#37396=CARTESIAN_POINT('Ctrl Pts',(-0.039384578838078,-0.151609390787265,
-5.55933009525148E-18));
#37397=CARTESIAN_POINT('Ctrl Pts',(-0.0319621170202007,-0.152230829911641,
-1.73472347597681E-18));
#37398=CARTESIAN_POINT('Ctrl Pts',(-0.195258838497135,0.000160033407109407,
-0.0621869692124234));
#37399=CARTESIAN_POINT('Ctrl Pts',(-0.194908302996182,-0.0446298405868324,
-0.0596372316287988));
#37400=CARTESIAN_POINT('Ctrl Pts',(-0.179587999130102,-0.0896361310987459,
-0.0570874940451742));
#37401=CARTESIAN_POINT('Ctrl Pts',(-0.151367887745159,-0.124066604758376,
-0.0545377564615496));
#37402=CARTESIAN_POINT('Ctrl Pts',(-0.110498449726745,-0.173930125493011,
-0.0508451295716089));
#37403=CARTESIAN_POINT('Ctrl Pts',(-0.0425730413282883,-0.201611998394397,
-0.047152502681668));
#37404=CARTESIAN_POINT('Ctrl Pts',(0.0215115638128062,-0.194527267086113,
-0.0434598757917273));
#37405=CARTESIAN_POINT('Ctrl Pts',(0.0855961689539017,-0.187442535777828,
-0.0397672489017865));
#37406=CARTESIAN_POINT('Ctrl Pts',(0.145839970837636,-0.145591200259874,
-0.0360746220118458));
#37407=CARTESIAN_POINT('Ctrl Pts',(0.17482372188203,-0.0879965379466177,
-0.032381995121905));
#37408=CARTESIAN_POINT('Ctrl Pts',(0.203807472926425,-0.0304018756333616,
-0.0286893682319642));
#37409=CARTESIAN_POINT('Ctrl Pts',(0.201531173131478,0.0429361134751947,
-0.0249967413420234));
#37410=CARTESIAN_POINT('Ctrl Pts',(0.169051968254342,0.0986198088313519,
-0.0213041144520826));
#37411=CARTESIAN_POINT('Ctrl Pts',(0.136572763377205,0.154303504187508,
-0.0176114875621418));
#37412=CARTESIAN_POINT('Ctrl Pts',(0.0738906534178767,0.192332905791266,
-0.013918860672201));
#37413=CARTESIAN_POINT('Ctrl Pts',(0.00948164844188619,0.19546885952366,
-0.0102262337822603));
#37414=CARTESIAN_POINT('Ctrl Pts',(-0.0499757118780851,0.198363726958473,
-0.00681748918817344));
#37415=CARTESIAN_POINT('Ctrl Pts',(-0.110904652631899,0.171524004472446,
-0.00340874459408663));
#37416=CARTESIAN_POINT('Ctrl Pts',(-0.14957294282862,0.126218275177078,
2.60208521396521E-16));
#37417=CARTESIAN_POINT('',(-0.0903606778650212,-0.126612599672283,-0.7746));
#37418=CARTESIAN_POINT('Ctrl Pts',(-0.0905528965052105,-0.126780367713603,
-0.7746));
#37419=CARTESIAN_POINT('Ctrl Pts',(-0.0940851012826834,-0.124893446464691,
-0.7746));
#37420=CARTESIAN_POINT('Ctrl Pts',(-0.0975325099084221,-0.122865237059866,
-0.7746));
#37421=CARTESIAN_POINT('Ctrl Pts',(-0.100885595415379,-0.120697716718052,
-0.7746));
#37422=CARTESIAN_POINT('Ctrl Pts',(-0.108471912208483,-0.115793727262852,
-0.7746));
#37423=CARTESIAN_POINT('Ctrl Pts',(-0.115576183595968,-0.11017842588183,
-0.7746));
#37424=CARTESIAN_POINT('Ctrl Pts',(-0.122169299632121,-0.103959921816958,
-0.7746));
#37425=CARTESIAN_POINT('Ctrl Pts',(-0.124862496418268,-0.101419748844069,
-0.7746));
#37426=CARTESIAN_POINT('Ctrl Pts',(-0.127468591019258,-0.0987799359225111,
-0.7746));
#37427=CARTESIAN_POINT('Ctrl Pts',(-0.129979488448584,-0.0960543571919703,
-0.7746));
#37428=CARTESIAN_POINT('Ctrl Pts',(-0.135808916607278,-0.0897265139216807,
-0.7746));
#37429=CARTESIAN_POINT('Ctrl Pts',(-0.141135846833842,-0.0829282927568507,
-0.7746));
#37430=CARTESIAN_POINT('Ctrl Pts',(-0.145934371304684,-0.0757454531871112,
-0.7746));
#37431=CARTESIAN_POINT('Ctrl Pts',(-0.149045007814598,-0.0710891878817545,
-0.7746));
#37432=CARTESIAN_POINT('Ctrl Pts',(-0.151935890614529,-0.0662652353489526,
-0.7746));
#37433=CARTESIAN_POINT('Ctrl Pts',(-0.154582417168357,-0.0613252527221335,
-0.7746));
#37434=CARTESIAN_POINT('Ctrl Pts',(-0.160106278576474,-0.0510144627738566,
-0.7746));
#37435=CARTESIAN_POINT('Ctrl Pts',(-0.164582453970299,-0.0401834658705794,
-0.7746));
#37436=CARTESIAN_POINT('Ctrl Pts',(-0.167945042441492,-0.0290261639881964,
-0.7746));
#37437=CARTESIAN_POINT('Ctrl Pts',(-0.169541196767554,-0.0237300131748207,
-0.7746));
#37438=CARTESIAN_POINT('Ctrl Pts',(-0.170885936193958,-0.0183597450823107,
-0.7746));
#37439=CARTESIAN_POINT('Ctrl Pts',(-0.171968925586268,-0.0129337153015973,
-0.7746));
#37440=CARTESIAN_POINT('Ctrl Pts',(-0.172843537099442,-0.00855170736067374,
-0.7746));
#37441=CARTESIAN_POINT('Ctrl Pts',(-0.173547366331531,-0.0041299597130302,
-0.7746));
#37442=CARTESIAN_POINT('Ctrl Pts',(-0.174071922613245,0.000296384781912512,
-0.7746));
#37443=CARTESIAN_POINT('Ctrl Pts',(-0.17489447630929,0.00723731019107897,
-0.7746));
#37444=CARTESIAN_POINT('Ctrl Pts',(-0.175279511390988,0.0142012653081574,
-0.7746));
#37445=CARTESIAN_POINT('Ctrl Pts',(-0.175212365254669,0.0211498412838069,
-0.7746));
#37446=CARTESIAN_POINT('Ctrl Pts',(-0.175138215020913,0.0288232319077874,
-0.7746));
#37447=CARTESIAN_POINT('Ctrl Pts',(-0.174512946184563,0.0364780095010279,
-0.7746));
#37448=CARTESIAN_POINT('Ctrl Pts',(-0.173371562479243,0.0440753847157037,
-0.7746));
#37449=CARTESIAN_POINT('Ctrl Pts',(-0.172636569880567,0.0489677049110253,
-0.7746));
#37450=CARTESIAN_POINT('Ctrl Pts',(-0.171687349129919,0.0538362733301391,
-0.7746));
#37451=CARTESIAN_POINT('Ctrl Pts',(-0.170531114314323,0.0586708415584075,
-0.7746));
#37452=CARTESIAN_POINT('Ctrl Pts',(-0.169750782077226,0.0619336471668159,
-0.7746));
#37453=CARTESIAN_POINT('Ctrl Pts',(-0.168876703665589,0.0651778442623389,
-0.7746));
#37454=CARTESIAN_POINT('Ctrl Pts',(-0.167914250210792,0.0683919284573595,
-0.7746));
#37455=CARTESIAN_POINT('Ctrl Pts',(-0.164635838743272,0.0793400843707924,
-0.7746));
#37456=CARTESIAN_POINT('Ctrl Pts',(-0.160328586154646,0.0899671574594893,
-0.7746));
#37457=CARTESIAN_POINT('Ctrl Pts',(-0.155100469158035,0.100152140039335,
-0.7746));
#37458=CARTESIAN_POINT('Ctrl Pts',(-0.151778955638379,0.106622836345163,
-0.7746));
#37459=CARTESIAN_POINT('Ctrl Pts',(-0.148084885651745,0.112915234045713,
-0.7746));
#37460=CARTESIAN_POINT('Ctrl Pts',(-0.144037924095902,0.118997135380321,
-0.7746));
#37461=CARTESIAN_POINT('Ctrl Pts',(-0.141313178735255,0.123091968557436,
-0.7746));
#37462=CARTESIAN_POINT('Ctrl Pts',(-0.138425284714667,0.127094620860079,
-0.7746));
#37463=CARTESIAN_POINT('Ctrl Pts',(-0.135397693361022,0.130972343961411,
-0.7746));
#37464=CARTESIAN_POINT('Ctrl Pts',(-0.127505121547234,0.141081108479578,
-0.7746));
#37465=CARTESIAN_POINT('Ctrl Pts',(-0.118649514256097,0.150371904390044,
-0.7746));
#37466=CARTESIAN_POINT('Ctrl Pts',(-0.108949064714297,0.158681874715884,
-0.7746));
#37467=CARTESIAN_POINT('Ctrl Pts',(-0.101799585751722,0.164806534997679,
-0.7746));
#37468=CARTESIAN_POINT('Ctrl Pts',(-0.0941900010005582,0.170398440943833,
-0.7746));
#37469=CARTESIAN_POINT('Ctrl Pts',(-0.0861525859670496,0.175382131162756,
-0.7746));
#37470=CARTESIAN_POINT('Ctrl Pts',(-0.0905528965052109,-0.126780367713602,
-0.7746));
#37471=CARTESIAN_POINT('Ctrl Pts',(-0.0518141871612445,-0.154123000442621,
-0.771191255405913));
#37472=CARTESIAN_POINT('Ctrl Pts',(0.0570960259948757,-0.17228938136959,
-0.764089883921885));
#37473=CARTESIAN_POINT('Ctrl Pts',(0.176570107319903,-0.0505019485347378,
-0.753295885547919));
#37474=CARTESIAN_POINT('Ctrl Pts',(0.138565293653093,0.120555556476704,
-0.742218004878094));
#37475=CARTESIAN_POINT('Ctrl Pts',(-0.0255413571731973,0.181859045827175,
-0.731140124208274));
#37476=CARTESIAN_POINT('Ctrl Pts',(-0.140076662830731,0.0971797286032077,
-0.722132248395451));
#37477=CARTESIAN_POINT('Ctrl Pts',(-0.155378700824008,0.0227870178177375,
-0.71681699947257));
#37478=CARTESIAN_POINT('Ctrl Pts',(-0.155313284670072,5.07842058496948E-5,
-0.71519437743963));
#37479=CARTESIAN_POINT('Origin',(-2.59090492670967E-17,0.,-0.7746));
#37480=CARTESIAN_POINT('',(-0.1954,-2.39295984553393E-17,-0.7746));
#37481=CARTESIAN_POINT('Origin',(0.,0.,-0.7746));
#37482=CARTESIAN_POINT('Origin',(0.,0.,-0.7746));
#37483=CARTESIAN_POINT('',(0.0903606778650188,-0.126612599672285,-0.7746));
#37484=CARTESIAN_POINT('Ctrl Pts',(0.0863566189666514,0.175629287040325,
-0.7746));
#37485=CARTESIAN_POINT('Ctrl Pts',(0.0905917700201877,0.173030418616691,
-0.7746));
#37486=CARTESIAN_POINT('Ctrl Pts',(0.0947139527180262,0.17026341030673,
-0.7746));
#37487=CARTESIAN_POINT('Ctrl Pts',(0.0987115944104381,0.167327732998805,
-0.7746));
#37488=CARTESIAN_POINT('Ctrl Pts',(0.105953907859282,0.162009323575319,
-0.7746));
#37489=CARTESIAN_POINT('Ctrl Pts',(0.112788112244188,0.156137654118489,
-0.7746));
#37490=CARTESIAN_POINT('Ctrl Pts',(0.119181447487494,0.149778658377445,
-0.7746));
#37491=CARTESIAN_POINT('Ctrl Pts',(0.123531334816534,0.145452134904685,
-0.7746));
#37492=CARTESIAN_POINT('Ctrl Pts',(0.127679589020936,0.14089585436879,-0.7746));
#37493=CARTESIAN_POINT('Ctrl Pts',(0.131595286168026,0.136152923130775,
-0.7746));
#37494=CARTESIAN_POINT('Ctrl Pts',(0.136118691747208,0.130673898370227,
-0.7746));
#37495=CARTESIAN_POINT('Ctrl Pts',(0.14033725682518,0.124941332985309,-0.7746));
#37496=CARTESIAN_POINT('Ctrl Pts',(0.14423394336631,0.118987826111841,-0.7746));
#37497=CARTESIAN_POINT('Ctrl Pts',(0.147634565650473,0.113792225200879,
-0.7746));
#37498=CARTESIAN_POINT('Ctrl Pts',(0.150789992297107,0.108428273261232,
-0.7746));
#37499=CARTESIAN_POINT('Ctrl Pts',(0.153685759550622,0.102916971941204,
-0.7746));
#37500=CARTESIAN_POINT('Ctrl Pts',(0.155604519974895,0.0992651360257737,
-0.7746));
#37501=CARTESIAN_POINT('Ctrl Pts',(0.157404880950174,0.0955566958497009,
-0.7746));
#37502=CARTESIAN_POINT('Ctrl Pts',(0.159082343688173,0.0918015394804238,
-0.7746));
#37503=CARTESIAN_POINT('Ctrl Pts',(0.16405867800029,0.0806615522458402,
-0.7746));
#37504=CARTESIAN_POINT('Ctrl Pts',(0.167962220294764,0.06910108595545,-0.7746));
#37505=CARTESIAN_POINT('Ctrl Pts',(0.170688770138284,0.0572850954713528,
-0.7746));
#37506=CARTESIAN_POINT('Ctrl Pts',(0.172036365341412,0.0514450510891004,
-0.7746));
#37507=CARTESIAN_POINT('Ctrl Pts',(0.173095662873938,0.0455425323535238,
-0.7746));
#37508=CARTESIAN_POINT('Ctrl Pts',(0.173849202315553,0.0395981476128783,
-0.7746));
#37509=CARTESIAN_POINT('Ctrl Pts',(0.174321899067488,0.0358692235460382,
-0.7746));
#37510=CARTESIAN_POINT('Ctrl Pts',(0.174673965346606,0.0321229165232209,
-0.7746));
#37511=CARTESIAN_POINT('Ctrl Pts',(0.174900309122346,0.028380866512874,
-0.7746));
#37512=CARTESIAN_POINT('Ctrl Pts',(0.175321177537221,0.0214228193958648,
-0.7746));
#37513=CARTESIAN_POINT('Ctrl Pts',(0.175309856312594,0.0144660238244896,
-0.7746));
#37514=CARTESIAN_POINT('Ctrl Pts',(0.174844198658199,0.00754289949041315,
-0.7746));
#37515=CARTESIAN_POINT('Ctrl Pts',(0.174292106830062,-0.000665277340672647,
-0.7746));
#37516=CARTESIAN_POINT('Ctrl Pts',(0.173101464382142,-0.00882644735382486,
-0.7746));
#37517=CARTESIAN_POINT('Ctrl Pts',(0.171304475172341,-0.016882029516175,
-0.7746));
#37518=CARTESIAN_POINT('Ctrl Pts',(0.170314958987332,-0.0213178541086821,
-0.7746));
#37519=CARTESIAN_POINT('Ctrl Pts',(0.169141391072696,-0.0257215634108893,
-0.7746));
#37520=CARTESIAN_POINT('Ctrl Pts',(0.167787923338702,-0.0300823658649688,
-0.7746));
#37521=CARTESIAN_POINT('Ctrl Pts',(0.166714256292423,-0.0335416650951491,
-0.7746));
#37522=CARTESIAN_POINT('Ctrl Pts',(0.165529733571263,-0.0369660268452503,
-0.7746));
#37523=CARTESIAN_POINT('Ctrl Pts',(0.164239345981684,-0.040346349804367,
-0.7746));
#37524=CARTESIAN_POINT('Ctrl Pts',(0.16079130903207,-0.0493788905376982,
-0.7746));
#37525=CARTESIAN_POINT('Ctrl Pts',(0.156585614990708,-0.0581084965167856,
-0.774600000000001));
#37526=CARTESIAN_POINT('Ctrl Pts',(0.151676017384677,-0.0664377067708377,
-0.774600000000001));
#37527=CARTESIAN_POINT('Ctrl Pts',(0.148484180335376,-0.0718527089794996,
-0.774600000000001));
#37528=CARTESIAN_POINT('Ctrl Pts',(0.144994377343054,-0.0770982050079457,
-0.7746));
#37529=CARTESIAN_POINT('Ctrl Pts',(0.141217726682289,-0.0821426785805183,
-0.7746));
#37530=CARTESIAN_POINT('Ctrl Pts',(0.138501407060657,-0.0857708676233492,
-0.7746));
#37531=CARTESIAN_POINT('Ctrl Pts',(0.135633582499286,-0.0892978390970129,
-0.7746));
#37532=CARTESIAN_POINT('Ctrl Pts',(0.132636760309005,-0.0926906541131664,
-0.7746));
#37533=CARTESIAN_POINT('Ctrl Pts',(0.125503512371863,-0.100766472155882,
-0.7746));
#37534=CARTESIAN_POINT('Ctrl Pts',(0.117625088446425,-0.108109649572534,
-0.7746));
#37535=CARTESIAN_POINT('Ctrl Pts',(0.109066551488383,-0.114565445008817,
-0.7746));
#37536=CARTESIAN_POINT('Ctrl Pts',(0.103151057383426,-0.119027565115719,
-0.7746));
#37537=CARTESIAN_POINT('Ctrl Pts',(0.0969100292154159,-0.123065020826135,
-0.7746));
#37538=CARTESIAN_POINT('Ctrl Pts',(0.0903606778650199,-0.126612599672284,
-0.7746));
#37539=CARTESIAN_POINT('Origin',(0.,0.,-0.7746));
#37540=CARTESIAN_POINT('Origin',(0.,0.,-0.90400562256037));
#37541=CARTESIAN_POINT('Ctrl Pts',(0.0903606778650188,-0.126612599672285,
-0.7746));
#37542=CARTESIAN_POINT('Ctrl Pts',(0.132326349903352,-0.0966626058939412,
-0.77090737311006));
#37543=CARTESIAN_POINT('Ctrl Pts',(0.183438243169013,0.00770935888928891,
-0.763522119330179));
#37544=CARTESIAN_POINT('Ctrl Pts',(0.0933467737565466,0.158298955986194,
-0.752444238660355));
#37545=CARTESIAN_POINT('Ctrl Pts',(-0.0817572628182647,0.164390938130267,
-0.741366357990534));
#37546=CARTESIAN_POINT('Ctrl Pts',(-0.152758625409659,0.0633569399596061,
-0.733553485957205));
#37547=CARTESIAN_POINT('Ctrl Pts',(-0.155762614151669,0.00605970375071522,
-0.729433240813817));
#37548=CARTESIAN_POINT('Ctrl Pts',(-0.155718793124499,0.000108222005882058,
-0.72900562256037));
#37549=CARTESIAN_POINT('Ctrl Pts',(0.113509973994371,-0.159049193030953,
-0.797607408227207));
#37550=CARTESIAN_POINT('Ctrl Pts',(0.166226735912021,-0.12142637860287,
-0.793914781337266));
#37551=CARTESIAN_POINT('Ctrl Pts',(0.230432868628899,0.0096844019734276,
-0.786529527557385));
#37552=CARTESIAN_POINT('Ctrl Pts',(0.117261070987011,0.198853204755397,
-0.775451646887562));
#37553=CARTESIAN_POINT('Ctrl Pts',(-0.102702469654057,0.206505877921275,
-0.76437376621774));
#37554=CARTESIAN_POINT('Ctrl Pts',(-0.229166552539487,0.026549163675777,
-0.753295885547918));
#37555=CARTESIAN_POINT('Ctrl Pts',(-0.147138184514376,-0.177715596359759,
-0.742218004878095));
#37556=CARTESIAN_POINT('Ctrl Pts',(0.0687852681232544,-0.220197695999892,
-0.731140124208273));
#37557=CARTESIAN_POINT('Ctrl Pts',(0.222113639748162,-0.0623631311604367,
-0.720062243538451));
#37558=CARTESIAN_POINT('Ctrl Pts',(0.173344387514496,0.152237478465231,
-0.708984362868628));
#37559=CARTESIAN_POINT('Ctrl Pts',(-0.0331531249511722,0.228305613963639,
-0.697906482198806));
#37560=CARTESIAN_POINT('Ctrl Pts',(-0.20948351797168,0.0966442108510496,
-0.686828601528984));
#37561=CARTESIAN_POINT('Ctrl Pts',(-0.195205176657611,-0.122957014602741,
-0.675750720859161));
#37562=CARTESIAN_POINT('Ctrl Pts',(-0.0033091362147546,-0.230677863194179,
-0.664672840189339));
#37563=CARTESIAN_POINT('Ctrl Pts',(0.191597738574492,-0.128505532717413,
-0.653594959519517));
#37564=CARTESIAN_POINT('Ctrl Pts',(0.212169696530742,0.0905945808558615,
-0.642517078849694));
#37565=CARTESIAN_POINT('Ctrl Pts',(0.0396881681025756,0.22726234506108,
-0.631439198179872));
#37566=CARTESIAN_POINT('Ctrl Pts',(-0.168905646876196,0.15714397242725,
-0.62036131751005));
#37567=CARTESIAN_POINT('Ctrl Pts',(-0.223812036237873,-0.055959942437397,
-0.609283436840227));
#37568=CARTESIAN_POINT('Ctrl Pts',(-0.0750715971962314,-0.218145808496258,
-0.598205556170405));
#37569=CARTESIAN_POINT('Ctrl Pts',(0.141976568990925,-0.181840577314685,
-0.587127675500583));
#37570=CARTESIAN_POINT('Ctrl Pts',(0.229840097781903,0.0199216082515445,
-0.576049794830761));
#37571=CARTESIAN_POINT('Ctrl Pts',(0.10857186341542,0.203557095173597,-0.564971914160938));
#37572=CARTESIAN_POINT('Ctrl Pts',(-0.111486030559036,0.201975755934477,
-0.553894033491116));
#37573=CARTESIAN_POINT('Ctrl Pts',(-0.230102660760181,0.0166164488813726,
-0.542816152821293));
#37574=CARTESIAN_POINT('Ctrl Pts',(-0.139348622206933,-0.183862182889048,
-0.531738272151472));
#37575=CARTESIAN_POINT('Ctrl Pts',(0.0781988836276648,-0.217044408992555,
-0.520660391481649));
#37576=CARTESIAN_POINT('Ctrl Pts',(0.22459313774015,-0.0527376841718607,
-0.509582510811826));
#37577=CARTESIAN_POINT('Ctrl Pts',(0.166629844370711,0.159555118412653,
-0.498504630142004));
#37578=CARTESIAN_POINT('Ctrl Pts',(-0.0429501309254399,0.226668540185073,
-0.487426749472182));
#37579=CARTESIAN_POINT('Ctrl Pts',(-0.213449734014577,0.0875360034570956,
-0.476348868802359));
#37580=CARTESIAN_POINT('Ctrl Pts',(-0.18973118516252,-0.131245640798648,
-0.465270988132538));
#37581=CARTESIAN_POINT('Ctrl Pts',(0.00662398147309128,-0.230606729569085,
-0.454193107462714));
#37582=CARTESIAN_POINT('Ctrl Pts',(0.196951979951472,-0.120138496934387,
-0.443115226792893));
#37583=CARTESIAN_POINT('Ctrl Pts',(0.208073151382307,0.0996438885547388,
-0.43203734612307));
#37584=CARTESIAN_POINT('Ctrl Pts',(0.0298683294310498,0.22876018829691,
-0.420959465453248));
#37585=CARTESIAN_POINT('Ctrl Pts',(-0.175513718907489,0.149727336608304,
-0.409881584783426));
#37586=CARTESIAN_POINT('Ctrl Pts',(-0.221195637922984,-0.0655425862808919,
-0.398803704113603));
#37587=CARTESIAN_POINT('Ctrl Pts',(-0.0656113983622211,-0.2211752365377,
-0.387725823443782));
#37588=CARTESIAN_POINT('Ctrl Pts',(0.149672726021042,-0.175560291461564,
-0.376647942773958));
#37589=CARTESIAN_POINT('Ctrl Pts',(0.228769469437527,0.0297971593569934,
-0.365570062104137));
#37590=CARTESIAN_POINT('Ctrl Pts',(0.0997086165043611,0.208042141517638,
-0.354492181434313));
#37591=CARTESIAN_POINT('Ctrl Pts',(-0.120077218212226,0.19698934620816,
-0.343414300764492));
#37592=CARTESIAN_POINT('Ctrl Pts',(-0.230604657647227,0.0066957242496528,
-0.33233642009467));
#37593=CARTESIAN_POINT('Ctrl Pts',(-0.131304660930752,-0.189690344693647,
-0.321258539424847));
#37594=CARTESIAN_POINT('Ctrl Pts',(0.0874695937736782,-0.21347695665156,
-0.310180658755026));
#37595=CARTESIAN_POINT('Ctrl Pts',(0.22665516716062,-0.0430206467417004,
-0.299102778085202));
#37596=CARTESIAN_POINT('Ctrl Pts',(0.159606950243788,0.16658019775968,-0.288024897415381));
#37597=CARTESIAN_POINT('Ctrl Pts',(-0.0526678094533962,0.22460953390923,
-0.276947016745558));
#37598=CARTESIAN_POINT('Ctrl Pts',(-0.217020070229199,0.0782664035548432,
-0.265869136075736));
#37599=CARTESIAN_POINT('Ctrl Pts',(-0.183905526410112,-0.139291414732429,
-0.254791255405913));
#37600=CARTESIAN_POINT('Ctrl Pts',(0.0165448622730762,-0.230107819353187,
-0.243713374736092));
#37601=CARTESIAN_POINT('Ctrl Pts',(0.201941061299588,-0.111548860515046,
-0.232635494066268));
#37602=CARTESIAN_POINT('Ctrl Pts',(0.20359086438931,0.10850852943864,-0.221557613396447));
#37603=CARTESIAN_POINT('Ctrl Pts',(0.0199931085929222,0.229833890689264,
-0.210479732726624));
#37604=CARTESIAN_POINT('Ctrl Pts',(-0.181796392508897,0.142033130433819,
-0.199401852056802));
#37605=CARTESIAN_POINT('Ctrl Pts',(-0.218169165091539,-0.0750037207463776,
-0.188323971386979));
#37606=CARTESIAN_POINT('Ctrl Pts',(-0.0560295462102443,-0.223794628104333,
-0.177246090717157));
#37607=CARTESIAN_POINT('Ctrl Pts',(0.157091373949139,-0.168954503937514,
-0.166168210047335));
#37608=CARTESIAN_POINT('Ctrl Pts',(0.22727476385837,0.0396174193949855,
-0.155090329377513));
#37609=CARTESIAN_POINT('Ctrl Pts',(0.0906604263794466,0.212141585867888,
-0.14401244870769));
#37610=CARTESIAN_POINT('Ctrl Pts',(-0.128445619592358,0.191637547881033,
-0.132934568037868));
#37611=CARTESIAN_POINT('Ctrl Pts',(-0.230679452575857,-0.00323706553079172,
-0.121856687368046));
#37612=CARTESIAN_POINT('Ctrl Pts',(-0.123016650143841,-0.195167496218507,
-0.110778806698223));
#37613=CARTESIAN_POINT('Ctrl Pts',(0.096576961801934,-0.209512466241152,
-0.0997009260284009));
#37614=CARTESIAN_POINT('Ctrl Pts',(0.228299237964294,-0.0332262618594141,
-0.0886230453585787));
#37615=CARTESIAN_POINT('Ctrl Pts',(0.152283875490699,0.173301039684831,
-0.0775451646887562));
#37616=CARTESIAN_POINT('Ctrl Pts',(-0.0622796920736053,0.222125366380487,
-0.066467284018934));
#37617=CARTESIAN_POINT('Ctrl Pts',(-0.220203600073336,0.0688683747915814,
-0.0553894033491115));
#37618=CARTESIAN_POINT('Ctrl Pts',(-0.177709301322904,-0.147110744400408,
-0.0443115226792893));
#37619=CARTESIAN_POINT('Ctrl Pts',(0.0263784818207279,-0.229121475610455,
-0.0332336420094669));
#37620=CARTESIAN_POINT('Ctrl Pts',(0.206664974128708,-0.102870521914166,
-0.0221557613396446));
#37621=CARTESIAN_POINT('Ctrl Pts',(0.198510833186043,0.117416113433844,
-0.0110778806698224));
#37622=CARTESIAN_POINT('Ctrl Pts',(0.0732416199231106,0.192383362751592,
-0.00369262688994078));
#37623=CARTESIAN_POINT('Ctrl Pts',(0.00853826423430079,0.19521336543348,
0.));
#37624=CARTESIAN_POINT('Ctrl Pts',(0.105793541951254,-0.14823699524473,
-0.789938272151471));
#37625=CARTESIAN_POINT('Ctrl Pts',(0.154926607242464,-0.113171787699894,
-0.786245645261531));
#37626=CARTESIAN_POINT('Ctrl Pts',(0.214767993475604,0.00902605427871468,
-0.778860391481649));
#37627=CARTESIAN_POINT('Ctrl Pts',(0.109289638576856,0.185335121832329,
-0.767782510811827));
#37628=CARTESIAN_POINT('Ctrl Pts',(-0.0957207340421262,0.192467564657606,
-0.756704630142005));
#37629=CARTESIAN_POINT('Ctrl Pts',(-0.213587761821816,0.0247443459131021,
-0.745626749472182));
#37630=CARTESIAN_POINT('Ctrl Pts',(-0.137135699606669,-0.165634452526706,
-0.73454886880236));
#37631=CARTESIAN_POINT('Ctrl Pts',(0.0641092310459577,-0.205228610046981,
-0.723470988132537));
#37632=CARTESIAN_POINT('Ctrl Pts',(0.207014307533962,-0.0581236723123581,
-0.712393107462715));
#37633=CARTESIAN_POINT('Ctrl Pts',(0.161560399383393,0.141888342476082,
-0.701315226792893));
#37634=CARTESIAN_POINT('Ctrl Pts',(-0.0308993685040486,0.21278535003247,
-0.69023734612307));
#37635=CARTESIAN_POINT('Ctrl Pts',(-0.195242784107519,0.0900743169540612,
-0.679159465453249));
#37636=CARTESIAN_POINT('Ctrl Pts',(-0.181935087456304,-0.114598370740716,
-0.668081584783425));
#37637=CARTESIAN_POINT('Ctrl Pts',(-0.00308418043488711,-0.214996333258512,
-0.657003704113604));
#37638=CARTESIAN_POINT('Ctrl Pts',(0.178572883777165,-0.119769699420263,
-0.645925823443782));
#37639=CARTESIAN_POINT('Ctrl Pts',(0.197746355679923,0.0844359420856367,
-0.634847942773959));
#37640=CARTESIAN_POINT('Ctrl Pts',(0.0369901580396483,0.211813002770593,
-0.623770062104137));
#37641=CARTESIAN_POINT('Ctrl Pts',(-0.15742340527262,0.146461291940682,
-0.612692181434314));
#37642=CARTESIAN_POINT('Ctrl Pts',(-0.208597246671037,-0.0521557737131904,
-0.601614300764492));
#37643=CARTESIAN_POINT('Ctrl Pts',(-0.0699682141387932,-0.203316210289885,
-0.590536420094669));
#37644=CARTESIAN_POINT('Ctrl Pts',(0.132324971798349,-0.169479016403749,
-0.579458539424848));
#37645=CARTESIAN_POINT('Ctrl Pts',(0.214215519316177,0.0185673331085495,
-0.568380658755025));
#37646=CARTESIAN_POINT('Ctrl Pts',(0.101191125174026,0.189719240784877,
-0.557302778085203));
#37647=CARTESIAN_POINT('Ctrl Pts',(-0.103907186618782,0.188245401321736,
-0.546224897415381));
#37648=CARTESIAN_POINT('Ctrl Pts',(-0.214460233207651,0.0154868591715072,
-0.535147016745558));
#37649=CARTESIAN_POINT('Ctrl Pts',(-0.129875673392626,-0.171363192803534,
-0.524069136075736));
#37650=CARTESIAN_POINT('Ctrl Pts',(0.0728829069770984,-0.202289684157425,
-0.512991255405913));
#37651=CARTESIAN_POINT('Ctrl Pts',(0.209325248727962,-0.0491525652461543,
-0.501913374736091));
#37652=CARTESIAN_POINT('Ctrl Pts',(0.155302312302862,0.148708527711963,
-0.490835494066269));
#37653=CARTESIAN_POINT('Ctrl Pts',(-0.0400303719398065,0.211259564875664,
-0.479757613396447));
#37654=CARTESIAN_POINT('Ctrl Pts',(-0.198939375944839,0.0815852874254244,
-0.468679732726624));
#37655=CARTESIAN_POINT('Ctrl Pts',(-0.176833219060973,-0.122323534374517,
-0.457601852056802));
#37656=CARTESIAN_POINT('Ctrl Pts',(0.0061736818113679,-0.214930035312299,
-0.446523971386979));
#37657=CARTESIAN_POINT('Ctrl Pts',(0.183563142692745,-0.111971456499662,
-0.435446090717158));
#37658=CARTESIAN_POINT('Ctrl Pts',(0.193928294537228,0.0928700759329271,
-0.424368210047335));
#37659=CARTESIAN_POINT('Ctrl Pts',(0.027837874078222,0.213209022306409,
-0.413290329377513));
#37660=CARTESIAN_POINT('Ctrl Pts',(-0.163582259169408,0.139548840593563,
-0.40221244870769));
#37661=CARTESIAN_POINT('Ctrl Pts',(-0.206158711667045,-0.0610869874011697,
-0.391134568037868));
#37662=CARTESIAN_POINT('Ctrl Pts',(-0.0611511216226529,-0.206139697172249,
-0.380056687368046));
#37663=CARTESIAN_POINT('Ctrl Pts',(0.139497942445576,-0.163625665711405,
-0.368978806698223));
#37664=CARTESIAN_POINT('Ctrl Pts',(0.213217672513124,0.0277715421608559,
-0.357900926028401));
#37665=CARTESIAN_POINT('Ctrl Pts',(0.0929304036628409,0.19389939272972,
-0.346823045358578));
#37666=CARTESIAN_POINT('Ctrl Pts',(-0.111914343517997,0.183597968783398,
-0.335745164688757));
#37667=CARTESIAN_POINT('Ctrl Pts',(-0.214928104240127,0.00624054749880152,
-0.324667284018934));
#37668=CARTESIAN_POINT('Ctrl Pts',(-0.122378542305555,-0.176795154935814,
-0.313589403349112));
#37669=CARTESIAN_POINT('Ctrl Pts',(0.0815233922863349,-0.1989647479812,
-0.302511522679289));
#37670=CARTESIAN_POINT('Ctrl Pts',(0.211247100952243,-0.0400960940759599,
-0.291433642009467));
#37671=CARTESIAN_POINT('Ctrl Pts',(0.148756836004253,0.155256040678952,
-0.280355761339645));
#37672=CARTESIAN_POINT('Ctrl Pts',(-0.0490874406258331,0.209340530281999,
-0.269277880669823));
#37673=CARTESIAN_POINT('Ctrl Pts',(-0.202266999948351,0.0729458368853433,
-0.2582));
#37674=CARTESIAN_POINT('Ctrl Pts',(-0.171403589822867,-0.129822354894342,
-0.247122119330178));
#37675=CARTESIAN_POINT('Ctrl Pts',(0.0154201390359869,-0.214465041118413,
-0.236044238660356));
#37676=CARTESIAN_POINT('Ctrl Pts',(0.188213065235466,-0.10396574538109,
-0.224966357990533));
#37677=CARTESIAN_POINT('Ctrl Pts',(0.189750714362162,0.101132096654386,
-0.213888477320711));
#37678=CARTESIAN_POINT('Ctrl Pts',(0.0186339728415945,0.214209734183008,
-0.202810596650889));
#37679=CARTESIAN_POINT('Ctrl Pts',(-0.169437835290407,0.13237768818239,
-0.191732715981066));
#37680=CARTESIAN_POINT('Ctrl Pts',(-0.203337979098878,-0.0699049519443599,
-0.180654835311244));
#37681=CARTESIAN_POINT('Ctrl Pts',(-0.052220645806835,-0.208581021946098,
-0.169576954641422));
#37682=CARTESIAN_POINT('Ctrl Pts',(0.14641226911824,-0.157468941020574,
-0.158499073971599));
#37683=CARTESIAN_POINT('Ctrl Pts',(0.211824577335415,0.0369242188441669,
-0.147421193301777));
#37684=CARTESIAN_POINT('Ctrl Pts',(0.084497311416599,0.197720155985876,
-0.136343312631954));
#37685=CARTESIAN_POINT('Ctrl Pts',(-0.119713859202124,0.178609986838626,
-0.125265431962133));
#37686=CARTESIAN_POINT('Ctrl Pts',(-0.214997814593688,-0.00301700913126643,
-0.11418755129231));
#37687=CARTESIAN_POINT('Ctrl Pts',(-0.114653952245116,-0.181899968541422,
-0.103109670622488));
#37688=CARTESIAN_POINT('Ctrl Pts',(0.0900116395095307,-0.195269764467508,
-0.0920317899526653));
#37689=CARTESIAN_POINT('Ctrl Pts',(0.21277940747491,-0.0309675335497962,
-0.0809539092828432));
#37690=CARTESIAN_POINT('Ctrl Pts',(0.141931585421943,0.161519998348358,
-0.0698760286130206));
#37691=CARTESIAN_POINT('Ctrl Pts',(-0.0580459054323005,0.207025236987341,
-0.0587981479431985));
#37692=CARTESIAN_POINT('Ctrl Pts',(-0.205234112760265,0.0641866881053908,
-0.047720267273376));
#37693=CARTESIAN_POINT('Ctrl Pts',(-0.165628585427786,-0.137110124877453,
-0.0366423866035538));
#37694=CARTESIAN_POINT('Ctrl Pts',(0.024585267046665,-0.213545749231955,
-0.0255645059337314));
#37695=CARTESIAN_POINT('Ctrl Pts',(0.192615845471205,-0.0958773620740437,
-0.0144866252639091));
#37696=CARTESIAN_POINT('Ctrl Pts',(0.185016024754682,0.109434141205358,
-0.00340874459408687));
#37697=CARTESIAN_POINT('Ctrl Pts',(0.068262639107798,0.179305101056521,
0.00397650918579475));
#37698=CARTESIAN_POINT('Ctrl Pts',(0.00795783122553719,0.181942719557458,
0.00766913607573553));
#37699=CARTESIAN_POINT('Ctrl Pts',(0.0980771099081362,-0.137424797458508,
-0.782269136075736));
#37700=CARTESIAN_POINT('Ctrl Pts',(0.143626478572908,-0.104917196796917,
-0.778576509185795));
#37701=CARTESIAN_POINT('Ctrl Pts',(0.199103118322308,0.00836770658400184,
-0.771191255405914));
#37702=CARTESIAN_POINT('Ctrl Pts',(0.101318206166701,0.171817038909262,
-0.76011337473609));
#37703=CARTESIAN_POINT('Ctrl Pts',(-0.0887389984301955,0.178429251393937,
-0.74903549406627));
#37704=CARTESIAN_POINT('Ctrl Pts',(-0.198008971104146,0.022939528150427,
-0.737957613396445));
#37705=CARTESIAN_POINT('Ctrl Pts',(-0.127133214698961,-0.153553308693652,
-0.726879732726626));
#37706=CARTESIAN_POINT('Ctrl Pts',(0.0594331939686611,-0.190259524094072,
-0.715801852056801));
#37707=CARTESIAN_POINT('Ctrl Pts',(0.191914975319761,-0.0538842134642793,
-0.70472397138698));
#37708=CARTESIAN_POINT('Ctrl Pts',(0.149776411252289,0.131539206486933,
-0.693646090717157));
#37709=CARTESIAN_POINT('Ctrl Pts',(-0.0286456120569251,0.197265086101302,
-0.682568210047335));
#37710=CARTESIAN_POINT('Ctrl Pts',(-0.181002050243358,0.0835044230570726,
-0.671490329377513));
#37711=CARTESIAN_POINT('Ctrl Pts',(-0.168664998254998,-0.106239726878691,
-0.66041244870769));
#37712=CARTESIAN_POINT('Ctrl Pts',(-0.0028592246550194,-0.199314803322844,
-0.649334568037868));
#37713=CARTESIAN_POINT('Ctrl Pts',(0.165548028979837,-0.111033866123113,
-0.638256687368046));
#37714=CARTESIAN_POINT('Ctrl Pts',(0.183323014829104,0.078277303315412,
-0.627178806698223));
#37715=CARTESIAN_POINT('Ctrl Pts',(0.0342921479767208,0.196363660480105,
-0.616100926028401));
#37716=CARTESIAN_POINT('Ctrl Pts',(-0.145941163669044,0.135778611454114,
-0.605023045358579));
#37717=CARTESIAN_POINT('Ctrl Pts',(-0.193382457104201,-0.0483516049889837,
-0.593945164688756));
#37718=CARTESIAN_POINT('Ctrl Pts',(-0.0648648310813553,-0.188486612083512,
-0.582867284018935));
#37719=CARTESIAN_POINT('Ctrl Pts',(0.122673374605773,-0.157117455492814,
-0.571789403349112));
#37720=CARTESIAN_POINT('Ctrl Pts',(0.19859094085045,0.0172130579655545,
-0.560711522679289));
#37721=CARTESIAN_POINT('Ctrl Pts',(0.0938103869326332,0.175881386396157,
-0.549633642009467));
#37722=CARTESIAN_POINT('Ctrl Pts',(-0.0963283426785271,0.174515046708994,
-0.538555761339645));
#37723=CARTESIAN_POINT('Ctrl Pts',(-0.19881780565512,0.0143572694616418,
-0.527477880669822));
#37724=CARTESIAN_POINT('Ctrl Pts',(-0.12040272457832,-0.15886420271802,
-0.516400000000001));
#37725=CARTESIAN_POINT('Ctrl Pts',(0.0675669303265321,-0.187534959322295,
-0.505322119330178));
#37726=CARTESIAN_POINT('Ctrl Pts',(0.194057359715773,-0.0455674463204479,
-0.494244238660356));
#37727=CARTESIAN_POINT('Ctrl Pts',(0.143974780235013,0.137861937011274,
-0.483166357990533));
#37728=CARTESIAN_POINT('Ctrl Pts',(-0.0371106129541729,0.195850589566256,
-0.472088477320711));
#37729=CARTESIAN_POINT('Ctrl Pts',(-0.1844290178751,0.075634571393753,-0.461010596650889));
#37730=CARTESIAN_POINT('Ctrl Pts',(-0.163935252959427,-0.113401427950385,
-0.449932715981066));
#37731=CARTESIAN_POINT('Ctrl Pts',(0.00572338214964429,-0.199253341055513,
-0.438854835311244));
#37732=CARTESIAN_POINT('Ctrl Pts',(0.170174305434017,-0.103804416064937,
-0.427776954641422));
#37733=CARTESIAN_POINT('Ctrl Pts',(0.17978343769215,0.0860962633111156,
-0.416699073971599));
#37734=CARTESIAN_POINT('Ctrl Pts',(0.0258074187253941,0.197657856315907,
-0.405621193301777));
#37735=CARTESIAN_POINT('Ctrl Pts',(-0.151650799431327,0.129370344578822,
-0.394543312631955));
#37736=CARTESIAN_POINT('Ctrl Pts',(-0.191121785411107,-0.0566313885214476,
-0.383465431962133));
#37737=CARTESIAN_POINT('Ctrl Pts',(-0.0566908448830847,-0.191104157806798,
-0.37238755129231));
#37738=CARTESIAN_POINT('Ctrl Pts',(0.12932315887011,-0.151691039961245,
-0.361309670622488));
#37739=CARTESIAN_POINT('Ctrl Pts',(0.19766587558872,0.0257459249647184,
-0.350231789952665));
#37740=CARTESIAN_POINT('Ctrl Pts',(0.0861521908213209,0.179756643941802,
-0.339153909282844));
#37741=CARTESIAN_POINT('Ctrl Pts',(-0.103751468823769,0.170206591358636,
-0.32807602861302));
#37742=CARTESIAN_POINT('Ctrl Pts',(-0.199251550833027,0.00578537074795013,
-0.316998147943199));
#37743=CARTESIAN_POINT('Ctrl Pts',(-0.113452423680357,-0.163899965177981,
-0.305920267273376));
#37744=CARTESIAN_POINT('Ctrl Pts',(0.0755771907989914,-0.184452539310841,
-0.294842386603554));
#37745=CARTESIAN_POINT('Ctrl Pts',(0.195839034743866,-0.0371715414102192,
-0.283764505933731));
#37746=CARTESIAN_POINT('Ctrl Pts',(0.137906721764718,0.143931883598223,
-0.272686625263909));
#37747=CARTESIAN_POINT('Ctrl Pts',(-0.04550707179827,0.194071526654768,
-0.261608744594087));
#37748=CARTESIAN_POINT('Ctrl Pts',(-0.187513929667502,0.0676252702158433,
-0.250530863924265));
#37749=CARTESIAN_POINT('Ctrl Pts',(-0.158901653235621,-0.120353295056254,
-0.239452983254442));
#37750=CARTESIAN_POINT('Ctrl Pts',(0.0142954157988977,-0.198822262883639,
-0.22837510258462));
#37751=CARTESIAN_POINT('Ctrl Pts',(0.174485069171344,-0.0963826302471343,
-0.217297221914798));
#37752=CARTESIAN_POINT('Ctrl Pts',(0.175910564335014,0.0937556638701326,
-0.206219341244975));
#37753=CARTESIAN_POINT('Ctrl Pts',(0.0172748370902665,0.198585577676752,
-0.195141460575153));
#37754=CARTESIAN_POINT('Ctrl Pts',(-0.157079278071916,0.12272224593096,
-0.184063579905331));
#37755=CARTESIAN_POINT('Ctrl Pts',(-0.188506793106217,-0.0648061831423422,
-0.172985699235508));
#37756=CARTESIAN_POINT('Ctrl Pts',(-0.0484117454034254,-0.193367415787862,
-0.161907818565686));
#37757=CARTESIAN_POINT('Ctrl Pts',(0.135733164287341,-0.145983378103634,
-0.150829937895864));
#37758=CARTESIAN_POINT('Ctrl Pts',(0.196374390812461,0.0342310182933485,
-0.139752057226041));
#37759=CARTESIAN_POINT('Ctrl Pts',(0.0783341964537513,0.183298726103865,
-0.128674176556219));
#37760=CARTESIAN_POINT('Ctrl Pts',(-0.11098209881189,0.165582425796218,
-0.117596295886397));
#37761=CARTESIAN_POINT('Ctrl Pts',(-0.199316176611518,-0.00279695273174133,
-0.106518415216575));
#37762=CARTESIAN_POINT('Ctrl Pts',(-0.106291254346392,-0.168632440864337,
-0.0954405345467521));
#37763=CARTESIAN_POINT('Ctrl Pts',(0.0834463172171277,-0.181027062693864,
-0.08436265387693));
#37764=CARTESIAN_POINT('Ctrl Pts',(0.197259576985525,-0.0287088052401784,
-0.0732847732071076));
#37765=CARTESIAN_POINT('Ctrl Pts',(0.131579295353188,0.149738957011886,
-0.0622068925372851));
#37766=CARTESIAN_POINT('Ctrl Pts',(-0.0538121187909959,0.191925107594194,
-0.051129011867463));
#37767=CARTESIAN_POINT('Ctrl Pts',(-0.190264625447194,0.0595050014192004,
-0.0400511311976405));
#37768=CARTESIAN_POINT('Ctrl Pts',(-0.153547869532668,-0.127109505354499,
-0.0289732505278182));
#37769=CARTESIAN_POINT('Ctrl Pts',(0.0227920522726021,-0.197970022853455,
-0.0178953698579958));
#37770=CARTESIAN_POINT('Ctrl Pts',(0.178566716813701,-0.088884202233921,
-0.00681748918817358));
#37771=CARTESIAN_POINT('Ctrl Pts',(0.17152121632332,0.101452168976872,0.00426039148164866));
#37772=CARTESIAN_POINT('Ctrl Pts',(0.0632836582924853,0.16622683936145,
0.0116456452615303));
#37773=CARTESIAN_POINT('Ctrl Pts',(0.0073773982167736,0.168672073681435,
0.0153382721514711));
#37774=CARTESIAN_POINT('Ctrl Pts',(0.0903606778650188,-0.126612599672285,
-0.7746));
#37775=CARTESIAN_POINT('Ctrl Pts',(0.132326349903352,-0.0966626058939412,
-0.77090737311006));
#37776=CARTESIAN_POINT('Ctrl Pts',(0.183438243169013,0.00770935888928891,
-0.763522119330179));
#37777=CARTESIAN_POINT('Ctrl Pts',(0.0933467737565466,0.158298955986194,
-0.752444238660355));
#37778=CARTESIAN_POINT('Ctrl Pts',(-0.0817572628182647,0.164390938130267,
-0.741366357990534));
#37779=CARTESIAN_POINT('Ctrl Pts',(-0.182430180386475,0.021134710387752,
-0.730288477320711));
#37780=CARTESIAN_POINT('Ctrl Pts',(-0.117130729791253,-0.141472164860598,
-0.719210596650888));
#37781=CARTESIAN_POINT('Ctrl Pts',(0.0547571568913644,-0.175290438141162,
-0.708132715981067));
#37782=CARTESIAN_POINT('Ctrl Pts',(0.176815643105561,-0.0496447546162005,
-0.697054835311244));
#37783=CARTESIAN_POINT('Ctrl Pts',(0.137992423121185,0.121190070497784,
-0.685976954641421));
#37784=CARTESIAN_POINT('Ctrl Pts',(-0.0263918556098016,0.181744822170133,
-0.6748990739716));
#37785=CARTESIAN_POINT('Ctrl Pts',(-0.166761316379197,0.0769345291600839,
-0.663821193301777));
#37786=CARTESIAN_POINT('Ctrl Pts',(-0.155394909053691,-0.0978810830166665,
-0.652743312631956));
#37787=CARTESIAN_POINT('Ctrl Pts',(-0.00263426887515189,-0.183633273387178,
-0.641665431962132));
#37788=CARTESIAN_POINT('Ctrl Pts',(0.15252317418251,-0.102298032825963,
-0.630587551292311));
#37789=CARTESIAN_POINT('Ctrl Pts',(0.168899673978284,0.0721186645451872,
-0.619509670622488));
#37790=CARTESIAN_POINT('Ctrl Pts',(0.0315941379137935,0.180914318189617,
-0.608431789952666));
#37791=CARTESIAN_POINT('Ctrl Pts',(-0.134458922065469,0.125095930967546,
-0.597353909282843));
#37792=CARTESIAN_POINT('Ctrl Pts',(-0.178167667537365,-0.0445474362647772,
-0.586276028613021));
#37793=CARTESIAN_POINT('Ctrl Pts',(-0.0597614480239172,-0.173657013877139,
-0.575198147943198));
#37794=CARTESIAN_POINT('Ctrl Pts',(0.113021777413197,-0.144755894581878,
-0.564120267273377));
#37795=CARTESIAN_POINT('Ctrl Pts',(0.182966362384724,0.0158587828225596,
-0.553042386603554));
#37796=CARTESIAN_POINT('Ctrl Pts',(0.0864296486912397,0.162043532007437,
-0.541964505933732));
#37797=CARTESIAN_POINT('Ctrl Pts',(-0.0887494987382724,0.160784692096253,
-0.53088662526391));
#37798=CARTESIAN_POINT('Ctrl Pts',(-0.18317537810259,0.0132276797517765,
-0.519808744594086));
#37799=CARTESIAN_POINT('Ctrl Pts',(-0.110929775764013,-0.146365212632506,
-0.508730863924265));
#37800=CARTESIAN_POINT('Ctrl Pts',(0.0622509536759654,-0.172780234487164,
-0.497652983254442));
#37801=CARTESIAN_POINT('Ctrl Pts',(0.178789470703585,-0.0419823273947417,
-0.48657510258462));
#37802=CARTESIAN_POINT('Ctrl Pts',(0.132647248167164,0.127015346310585,
-0.475497221914797));
#37803=CARTESIAN_POINT('Ctrl Pts',(-0.0341908539685392,0.180441614256847,
-0.464419341244976));
#37804=CARTESIAN_POINT('Ctrl Pts',(-0.169918659805362,0.069683855362082,
-0.453341460575152));
#37805=CARTESIAN_POINT('Ctrl Pts',(-0.15103728685788,-0.104479321526254,
-0.442263579905332));
#37806=CARTESIAN_POINT('Ctrl Pts',(0.00527308248792088,-0.183576646798727,
-0.431185699235508));
#37807=CARTESIAN_POINT('Ctrl Pts',(0.15678546817529,-0.0956373756302127,
-0.420107818565687));
#37808=CARTESIAN_POINT('Ctrl Pts',(0.165638580847071,0.079322450689304,
-0.409029937895864));
#37809=CARTESIAN_POINT('Ctrl Pts',(0.023776963372566,0.182106690325406,
-0.397952057226042));
#37810=CARTESIAN_POINT('Ctrl Pts',(-0.139719339693246,0.119191848564081,
-0.386874176556219));
#37811=CARTESIAN_POINT('Ctrl Pts',(-0.176084859155169,-0.0521757896417255,
-0.375796295886397));
#37812=CARTESIAN_POINT('Ctrl Pts',(-0.0522305681435164,-0.176068618441347,
-0.364718415216575));
#37813=CARTESIAN_POINT('Ctrl Pts',(0.119148375294644,-0.139756414211085,
-0.353640534546752));
#37814=CARTESIAN_POINT('Ctrl Pts',(0.182114078664316,0.023720307768581,
-0.34256265387693));
#37815=CARTESIAN_POINT('Ctrl Pts',(0.0793739779798006,0.165613895153883,
-0.331484773207108));
#37816=CARTESIAN_POINT('Ctrl Pts',(-0.0955885941295399,0.156815213933875,
-0.320406892537285));
#37817=CARTESIAN_POINT('Ctrl Pts',(-0.183574997425927,0.00533019399709877,
-0.309329011867463));
#37818=CARTESIAN_POINT('Ctrl Pts',(-0.10452630505516,-0.151004775420149,
-0.29825113119764));
#37819=CARTESIAN_POINT('Ctrl Pts',(0.0696309893116479,-0.169940330640481,
-0.287173250527819));
#37820=CARTESIAN_POINT('Ctrl Pts',(0.180430968535489,-0.0342469887444786,
-0.276095369857996));
#37821=CARTESIAN_POINT('Ctrl Pts',(0.127056607525184,0.132607726517495,
-0.265017489188174));
#37822=CARTESIAN_POINT('Ctrl Pts',(-0.0419267029707069,0.178802523027537,
-0.253939608518351));
#37823=CARTESIAN_POINT('Ctrl Pts',(-0.172760859386654,0.0623047035463433,
-0.242861727848529));
#37824=CARTESIAN_POINT('Ctrl Pts',(-0.146399716648376,-0.110884235218166,
-0.231783847178707));
#37825=CARTESIAN_POINT('Ctrl Pts',(0.0131706925618085,-0.183179484648865,
-0.220705966508885));
#37826=CARTESIAN_POINT('Ctrl Pts',(0.160757073107222,-0.0887995151131783,
-0.209628085839062));
#37827=CARTESIAN_POINT('Ctrl Pts',(0.162070414307866,0.0863792310858789,
-0.19855020516924));
#37828=CARTESIAN_POINT('Ctrl Pts',(0.0159157013389389,0.182961421170497,
-0.187472324499417));
#37829=CARTESIAN_POINT('Ctrl Pts',(-0.144720720853425,0.113066803679531,
-0.176394443829595));
#37830=CARTESIAN_POINT('Ctrl Pts',(-0.173675607113556,-0.0597074143403244,
-0.165316563159773));
#37831=CARTESIAN_POINT('Ctrl Pts',(-0.044602845000016,-0.178153809629627,
-0.15423868248995));
#37832=CARTESIAN_POINT('Ctrl Pts',(0.125054059456442,-0.134497815186694,
-0.143160801820128));
#37833=CARTESIAN_POINT('Ctrl Pts',(0.180924204289506,0.0315378177425299,
-0.132082921150306));
#37834=CARTESIAN_POINT('Ctrl Pts',(0.0721710814909035,0.168877296221853,
-0.121005040480484));
#37835=CARTESIAN_POINT('Ctrl Pts',(-0.102250338421656,0.15255486475381,
-0.109927159810661));
#37836=CARTESIAN_POINT('Ctrl Pts',(-0.183634538629348,-0.00257689633221619,
-0.098849279140839));
#37837=CARTESIAN_POINT('Ctrl Pts',(-0.0979285564476671,-0.155364913187252,
-0.0877713984710165));
#37838=CARTESIAN_POINT('Ctrl Pts',(0.0768809949247246,-0.16678436092022,
-0.0766935178011943));
#37839=CARTESIAN_POINT('Ctrl Pts',(0.181739746496141,-0.0264500769305604,
-0.0656156371313721));
#37840=CARTESIAN_POINT('Ctrl Pts',(0.121227005284432,0.137957915675413,
-0.0545377564615496));
#37841=CARTESIAN_POINT('Ctrl Pts',(-0.0495783321496912,0.176824978201047,
-0.0434598757917274));
#37842=CARTESIAN_POINT('Ctrl Pts',(-0.175295138134123,0.0548233147330098,
-0.0323819951219049));
#37843=CARTESIAN_POINT('Ctrl Pts',(-0.141467153637551,-0.117108885831544,
-0.0213041144520827));
#37844=CARTESIAN_POINT('Ctrl Pts',(0.0209988374985395,-0.182394296474955,
-0.0102262337822603));
#37845=CARTESIAN_POINT('Ctrl Pts',(0.164517588156196,-0.0818910423937984,
0.000851646887561965));
#37846=CARTESIAN_POINT('Ctrl Pts',(0.158026407891959,0.0934701967483867,
0.0119295275573842));
#37847=CARTESIAN_POINT('Ctrl Pts',(0.0583046774771726,0.153148577666378,
0.0193147813372658));
#37848=CARTESIAN_POINT('Ctrl Pts',(0.00679696520801,0.155401427805413,0.0230074082272066));
#37849=CARTESIAN_POINT('',(0.00853826423430079,0.19521336543348,0.));
#37850=CARTESIAN_POINT('Ctrl Pts',(0.133815347598873,-0.0797905857758447,
1.28369537222284E-16));
#37851=CARTESIAN_POINT('Ctrl Pts',(0.136293565210637,-0.0766448939156863,
1.28593437618207E-16));
#37852=CARTESIAN_POINT('Ctrl Pts',(0.138637419022965,-0.0734038133327389,
7.54322313592872E-17));
#37853=CARTESIAN_POINT('Ctrl Pts',(0.140838976075351,-0.0700729779668307,
7.63278329429795E-17));
#37854=CARTESIAN_POINT('Ctrl Pts',(0.145819973356658,-0.0625370016067841,
7.81008351086913E-17));
#37855=CARTESIAN_POINT('Ctrl Pts',(0.150074011938905,-0.054542919364199,
-1.3346458730469E-16));
#37856=CARTESIAN_POINT('Ctrl Pts',(0.153617808369117,-0.046201435097827,
-1.04083408558608E-16));
#37857=CARTESIAN_POINT('Ctrl Pts',(0.155065400881004,-0.0427940525351372,
-9.20815977376891E-17));
#37858=CARTESIAN_POINT('Ctrl Pts',(0.156393229106788,-0.0393303545681794,
2.29694749575199E-16));
#37859=CARTESIAN_POINT('Ctrl Pts',(0.157599445512596,-0.0358262975538223,
1.6306400674182E-16));
#37860=CARTESIAN_POINT('Ctrl Pts',(0.160399820179621,-0.0276912129640526,
8.37282249230137E-18));
#37861=CARTESIAN_POINT('Ctrl Pts',(0.162551197740732,-0.0193269206951015,
-2.31903545997953E-16));
#37862=CARTESIAN_POINT('Ctrl Pts',(0.164064259316912,-0.0108223648054157,
-2.81025203108243E-16));
#37863=CARTESIAN_POINT('Ctrl Pts',(0.165045137245379,-0.00530908544195027,
-3.12869478336516E-16));
#37864=CARTESIAN_POINT('Ctrl Pts',(0.165757428744978,0.000269613978694174,
-5.88307172475674E-18));
#37865=CARTESIAN_POINT('Ctrl Pts',(0.166199326803605,0.00585654216766985,
-3.46944695195361E-18));
#37866=CARTESIAN_POINT('Ctrl Pts',(0.167121638500691,0.0175173519831342,
1.56817273628343E-18));
#37867=CARTESIAN_POINT('Ctrl Pts',(0.166875568718661,0.029234254531895,
-1.25050453494893E-16));
#37868=CARTESIAN_POINT('Ctrl Pts',(0.165478560136187,0.0408032009544139,
-1.09287578986539E-16));
#37869=CARTESIAN_POINT('Ctrl Pts',(0.164815426560599,0.0462947612090889,
-1.01805240319898E-16));
#37870=CARTESIAN_POINT('Ctrl Pts',(0.163892264719358,0.0517533269403495,
-1.02393347651096E-16));
#37871=CARTESIAN_POINT('Ctrl Pts',(0.16270697339196,0.0571579380710028,
-9.0205620750794E-17));
#37872=CARTESIAN_POINT('Ctrl Pts',(0.161749752444841,0.0615226093258332,
-8.03630215373626E-17));
#37873=CARTESIAN_POINT('Ctrl Pts',(0.160620157616345,0.0658551527740701,
-8.55423955822509E-17));
#37874=CARTESIAN_POINT('Ctrl Pts',(0.159324513207994,0.0701199726232436,
-6.59194920871187E-17));
#37875=CARTESIAN_POINT('Ctrl Pts',(0.15729280825055,0.0768076529576913,
-3.51487419850738E-17));
#37876=CARTESIAN_POINT('Ctrl Pts',(0.154851112214637,0.0833408692938153,
-2.23469952887909E-17));
#37877=CARTESIAN_POINT('Ctrl Pts',(0.152001406717412,0.0896785574668918,
4.85722573273506E-17));
#37878=CARTESIAN_POINT('Ctrl Pts',(0.148854441839518,0.096677344572132,
1.26781386779886E-16));
#37879=CARTESIAN_POINT('Ctrl Pts',(0.145210141356519,0.103437941488835,
9.23711880014318E-17));
#37880=CARTESIAN_POINT('Ctrl Pts',(0.141116132135723,0.109938863795627,
1.56125112837913E-16));
#37881=CARTESIAN_POINT('Ctrl Pts',(0.13847980310281,0.114125119686566,1.97179324966914E-16));
#37882=CARTESIAN_POINT('Ctrl Pts',(0.135656780122337,0.118203658930518,
-1.03755060408231E-16));
#37883=CARTESIAN_POINT('Ctrl Pts',(0.132657783307425,0.122167988997596,
-5.55111512312578E-17));
#37884=CARTESIAN_POINT('Ctrl Pts',(0.130633788308025,0.124843478411871,
-2.29517865663081E-17));
#37885=CARTESIAN_POINT('Ctrl Pts',(0.128531392348119,0.127464306685902,
-6.25671501750493E-17));
#37886=CARTESIAN_POINT('Ctrl Pts',(0.126360131478195,0.13002209138432,-6.07153216591882E-17));
#37887=CARTESIAN_POINT('Ctrl Pts',(0.118964139957754,0.138734703582444,
-5.44074163354499E-17));
#37888=CARTESIAN_POINT('Ctrl Pts',(0.110754606049639,0.146740382010002,
7.59358561344913E-17));
#37889=CARTESIAN_POINT('Ctrl Pts',(0.101878988500282,0.153971613547104,
-1.90819582357449E-17));
#37890=CARTESIAN_POINT('Ctrl Pts',(0.0962401643390006,0.158565732534371,
-7.94483208514698E-17));
#37891=CARTESIAN_POINT('Ctrl Pts',(0.0903316376136661,0.16284704475175,
-2.22921060177516E-16));
#37892=CARTESIAN_POINT('Ctrl Pts',(0.0841843402892172,0.166793948755328,
-2.33320307518881E-16));
#37893=CARTESIAN_POINT('Ctrl Pts',(0.0800454559343232,0.169451340836512,
-2.40321966923358E-16));
#37894=CARTESIAN_POINT('Ctrl Pts',(0.0757941213185356,0.171958832063456,
-8.02031543966986E-17));
#37895=CARTESIAN_POINT('Ctrl Pts',(0.0714649579678027,0.174295835998696,
-8.28330459778925E-17));
#37896=CARTESIAN_POINT('Ctrl Pts',(0.0601793857165482,0.18038810478734,
-8.96888352027333E-17));
#37897=CARTESIAN_POINT('Ctrl Pts',(0.0483399292857095,0.185344713462473,
-1.08355695937117E-16));
#37898=CARTESIAN_POINT('Ctrl Pts',(0.0361201977079082,0.189063915695687,
-1.57859836313889E-16));
#37899=CARTESIAN_POINT('Ctrl Pts',(0.0271139376768322,0.191805064485021,
-1.94345675467512E-16));
#37900=CARTESIAN_POINT('Ctrl Pts',(0.0179000121429095,0.193873604321062,
-1.33645313566251E-16));
#37901=CARTESIAN_POINT('Ctrl Pts',(0.00853826423430357,0.19521336543348,
-1.57859836313889E-16));
#37902=CARTESIAN_POINT('Ctrl Pts',(0.00853826423430082,0.19521336543348,
-1.73472347597681E-18));
#37903=CARTESIAN_POINT('Ctrl Pts',(0.0732416199231104,0.192383362751592,
-0.00369262688994077));
#37904=CARTESIAN_POINT('Ctrl Pts',(0.135876226554577,0.154899738092718,
-0.00738525377988161));
#37905=CARTESIAN_POINT('Ctrl Pts',(0.168552553360754,0.0994434865386125,
-0.0110778806698224));
#37906=CARTESIAN_POINT('Ctrl Pts',(0.201228880166931,0.043987234984507,
-0.0147705075597632));
#37907=CARTESIAN_POINT('Ctrl Pts',(0.20394692714782,-0.0294416434648305,
-0.018463134449704));
#37908=CARTESIAN_POINT('Ctrl Pts',(0.175258201920267,-0.087197908305547,
-0.0221557613396447));
#37909=CARTESIAN_POINT('Ctrl Pts',(0.146569476692714,-0.144954173146263,
-0.0258483882295855));
#37910=CARTESIAN_POINT('Ctrl Pts',(0.0864739792567223,-0.187037824378359,
-0.0295410151195261));
#37911=CARTESIAN_POINT('Ctrl Pts',(0.022411600014787,-0.194411194792733,
-0.0332336420094669));
#37912=CARTESIAN_POINT('Ctrl Pts',(-0.0416507792271474,-0.201784565207106,
-0.0369262688994076));
#37913=CARTESIAN_POINT('Ctrl Pts',(-0.109680040275024,-0.174447654803758,
-0.0406188957893484));
#37914=CARTESIAN_POINT('Ctrl Pts',(-0.150777053924035,-0.124782679736753,
-0.0443115226792891));
#37915=CARTESIAN_POINT('Ctrl Pts',(-0.179348311665281,-0.0902548472409218,
-0.0468786920487183));
#37916=CARTESIAN_POINT('Ctrl Pts',(-0.194902573031226,-0.0449353295028645,
-0.0494458614181474));
#37917=CARTESIAN_POINT('Ctrl Pts',(-0.195265563427387,0.000160747932399612,
-0.0520130307875765));
#37918=CARTESIAN_POINT('Origin',(0.324759526419164,-0.1875,0.5));
#37919=CARTESIAN_POINT('',(0.324759526419164,-0.1875,0.475));
#37920=CARTESIAN_POINT('',(0.352933712456347,-0.188249288476161,0.45));
#37921=CARTESIAN_POINT('Ctrl Pts',(0.324759526419164,-0.1875,0.475));
#37922=CARTESIAN_POINT('Ctrl Pts',(0.33839219708232,-0.187862558940078,
0.463012481414242));
#37923=CARTESIAN_POINT('Ctrl Pts',(0.352933712456347,-0.188249288476161,
0.45));
#37924=CARTESIAN_POINT('',(0.324759526419164,-0.1875,0.015));
#37925=CARTESIAN_POINT('',(0.324759526419164,-0.1875,0.5));
#37926=CARTESIAN_POINT('',(0.352933712456347,-0.188249288476161,0.04));
#37927=CARTESIAN_POINT('Ctrl Pts',(0.352933712456347,-0.188249288476161,
0.04));
#37928=CARTESIAN_POINT('Ctrl Pts',(0.338392197082319,-0.187862558940078,
0.0269875185857579));
#37929=CARTESIAN_POINT('Ctrl Pts',(0.324759526419164,-0.1875,0.015));
#37930=CARTESIAN_POINT('',(0.352933712456347,-0.188249288476161,0.245));
#37931=CARTESIAN_POINT('Origin',(0.362615522993687,-0.249218744246926,0.5));
#37932=CARTESIAN_POINT('',(0.339495522292874,-0.211524916601068,0.45));
#37933=CARTESIAN_POINT('Ctrl Pts',(0.339495522292874,-0.211524916601068,
0.45));
#37934=CARTESIAN_POINT('Ctrl Pts',(0.331889847003218,-0.19912495964568,
0.463012481414243));
#37935=CARTESIAN_POINT('Ctrl Pts',(0.324759526419164,-0.1875,0.475));
#37936=CARTESIAN_POINT('',(0.339495522292874,-0.211524916601068,0.04));
#37937=CARTESIAN_POINT('',(0.339495522292874,-0.211524916601068,0.245));
#37938=CARTESIAN_POINT('Ctrl Pts',(0.324759526419164,-0.1875,0.015));
#37939=CARTESIAN_POINT('Ctrl Pts',(0.331889847003216,-0.199124959645677,
0.0269875185857545));
#37940=CARTESIAN_POINT('Ctrl Pts',(0.339495522292874,-0.211524916601068,
0.04));
#37941=CARTESIAN_POINT('Origin',(0.1875,-0.324759526419164,0.5));
#37942=CARTESIAN_POINT('',(0.1875,-0.324759526419164,0.475));
#37943=CARTESIAN_POINT('',(0.211524916601068,-0.339495522292874,0.45));
#37944=CARTESIAN_POINT('Ctrl Pts',(0.1875,-0.324759526419164,0.475));
#37945=CARTESIAN_POINT('Ctrl Pts',(0.199124959645676,-0.331889847003216,
0.463012481414246));
#37946=CARTESIAN_POINT('Ctrl Pts',(0.211524916601068,-0.339495522292874,
0.45));
#37947=CARTESIAN_POINT('',(0.1875,-0.324759526419164,0.0150000000000001));
#37948=CARTESIAN_POINT('',(0.1875,-0.324759526419164,0.5));
#37949=CARTESIAN_POINT('',(0.211524916601068,-0.339495522292874,0.04));
#37950=CARTESIAN_POINT('Ctrl Pts',(0.211524916601068,-0.339495522292874,
0.04));
#37951=CARTESIAN_POINT('Ctrl Pts',(0.19912495964567,-0.331889847003212,
0.0269875185857474));
#37952=CARTESIAN_POINT('Ctrl Pts',(0.1875,-0.324759526419164,0.0150000000000001));
#37953=CARTESIAN_POINT('',(0.211524916601068,-0.339495522292874,0.245));
#37954=CARTESIAN_POINT('Origin',(0.18942488259565,-0.397137525113939,0.5));
#37955=CARTESIAN_POINT('',(0.188249288476161,-0.352933712456347,0.45));
#37956=CARTESIAN_POINT('Ctrl Pts',(0.188249288476161,-0.352933712456347,
0.45));
#37957=CARTESIAN_POINT('Ctrl Pts',(0.187862558940078,-0.338392197082316,
0.463012481414245));
#37958=CARTESIAN_POINT('Ctrl Pts',(0.1875,-0.324759526419164,0.475));
#37959=CARTESIAN_POINT('',(0.188249288476161,-0.352933712456347,0.04));
#37960=CARTESIAN_POINT('',(0.188249288476161,-0.352933712456347,0.245));
#37961=CARTESIAN_POINT('Ctrl Pts',(0.1875,-0.324759526419164,0.0150000000000001));
#37962=CARTESIAN_POINT('Ctrl Pts',(0.187862558940078,-0.338392197082329,
0.0269875185857667));
#37963=CARTESIAN_POINT('Ctrl Pts',(0.188249288476161,-0.352933712456347,
0.04));
#37964=CARTESIAN_POINT('Origin',(-6.88863824520386E-17,-0.375,0.5));
#37965=CARTESIAN_POINT('',(-6.88863824520386E-17,-0.375,0.475));
#37966=CARTESIAN_POINT('',(0.013438190163473,-0.399774205077229,0.45));
#37967=CARTESIAN_POINT('Ctrl Pts',(-6.88863824520386E-17,-0.375,0.475));
#37968=CARTESIAN_POINT('Ctrl Pts',(0.00650235007909994,-0.386987518585756,
0.463012481414244));
#37969=CARTESIAN_POINT('Ctrl Pts',(0.013438190163473,-0.399774205077229,
0.45));
#37970=CARTESIAN_POINT('',(-6.88863824520386E-17,-0.375,0.015));
#37971=CARTESIAN_POINT('',(-6.88863824520386E-17,-0.375,0.5));
#37972=CARTESIAN_POINT('',(0.013438190163473,-0.399774205077229,0.04));
#37973=CARTESIAN_POINT('Ctrl Pts',(0.013438190163473,-0.399774205077229,
0.04));
#37974=CARTESIAN_POINT('Ctrl Pts',(0.00650235007910186,-0.38698751858576,
0.0269875185857598));
#37975=CARTESIAN_POINT('Ctrl Pts',(-6.88863824520386E-17,-0.375,0.015));
#37976=CARTESIAN_POINT('',(0.013438190163473,-0.399774205077229,0.245));
#37977=CARTESIAN_POINT('Origin',(-0.0345220021202517,-0.438643626842576,
0.5));
#37978=CARTESIAN_POINT('',(-0.013438190163473,-0.399774205077229,0.45));
#37979=CARTESIAN_POINT('Ctrl Pts',(-0.013438190163473,-0.399774205077229,
0.45));
#37980=CARTESIAN_POINT('Ctrl Pts',(-0.00650235007910025,-0.386987518585757,
0.463012481414243));
#37981=CARTESIAN_POINT('Ctrl Pts',(-6.88863824520386E-17,-0.375,0.475));
#37982=CARTESIAN_POINT('',(-0.013438190163473,-0.399774205077229,0.04));
#37983=CARTESIAN_POINT('',(-0.013438190163473,-0.399774205077229,0.245));
#37984=CARTESIAN_POINT('Ctrl Pts',(-6.88863824520386E-17,-0.375,0.015));
#37985=CARTESIAN_POINT('Ctrl Pts',(-0.00650235007910422,-0.386987518585764,
0.0269875185857641));
#37986=CARTESIAN_POINT('Ctrl Pts',(-0.013438190163473,-0.399774205077229,
0.04));
#37987=CARTESIAN_POINT('Origin',(-0.1875,-0.324759526419164,0.5));
#37988=CARTESIAN_POINT('',(-0.1875,-0.324759526419164,0.475));
#37989=CARTESIAN_POINT('',(-0.188249288476161,-0.352933712456347,0.45));
#37990=CARTESIAN_POINT('Ctrl Pts',(-0.1875,-0.324759526419164,0.475));
#37991=CARTESIAN_POINT('Ctrl Pts',(-0.187862558940078,-0.33839219708232,
0.463012481414242));
#37992=CARTESIAN_POINT('Ctrl Pts',(-0.188249288476161,-0.352933712456347,
0.45));
#37993=CARTESIAN_POINT('',(-0.1875,-0.324759526419164,0.015));
#37994=CARTESIAN_POINT('',(-0.1875,-0.324759526419164,0.5));
#37995=CARTESIAN_POINT('',(-0.188249288476161,-0.352933712456347,0.04));
#37996=CARTESIAN_POINT('Ctrl Pts',(-0.188249288476161,-0.352933712456347,
0.04));
#37997=CARTESIAN_POINT('Ctrl Pts',(-0.187862558940078,-0.338392197082319,
0.0269875185857579));
#37998=CARTESIAN_POINT('Ctrl Pts',(-0.1875,-0.324759526419164,0.015));
#37999=CARTESIAN_POINT('',(-0.188249288476161,-0.352933712456347,0.245));
#38000=CARTESIAN_POINT('Origin',(-0.249218744246926,-0.362615522993687,
0.5));
#38001=CARTESIAN_POINT('',(-0.211524916601068,-0.339495522292874,0.45));
#38002=CARTESIAN_POINT('Ctrl Pts',(-0.211524916601068,-0.339495522292874,
0.45));
#38003=CARTESIAN_POINT('Ctrl Pts',(-0.199124959645674,-0.331889847003215,
0.463012481414248));
#38004=CARTESIAN_POINT('Ctrl Pts',(-0.1875,-0.324759526419164,0.475));
#38005=CARTESIAN_POINT('',(-0.211524916601068,-0.339495522292874,0.04));
#38006=CARTESIAN_POINT('',(-0.211524916601068,-0.339495522292874,0.245));
#38007=CARTESIAN_POINT('Ctrl Pts',(-0.1875,-0.324759526419164,0.015));
#38008=CARTESIAN_POINT('Ctrl Pts',(-0.199124959645673,-0.331889847003214,
0.0269875185857501));
#38009=CARTESIAN_POINT('Ctrl Pts',(-0.211524916601068,-0.339495522292874,
0.04));
#38010=CARTESIAN_POINT('Origin',(-0.324759526419164,-0.1875,0.5));
#38011=CARTESIAN_POINT('',(-0.324759526419164,-0.1875,0.475));
#38012=CARTESIAN_POINT('',(-0.339495522292874,-0.211524916601068,0.45));
#38013=CARTESIAN_POINT('Ctrl Pts',(-0.324759526419164,-0.1875,0.475));
#38014=CARTESIAN_POINT('Ctrl Pts',(-0.331889847003216,-0.199124959645676,
0.463012481414247));
#38015=CARTESIAN_POINT('Ctrl Pts',(-0.339495522292874,-0.211524916601068,
0.45));
#38016=CARTESIAN_POINT('',(-0.324759526419164,-0.1875,0.0150000000000001));
#38017=CARTESIAN_POINT('',(-0.324759526419164,-0.1875,0.5));
#38018=CARTESIAN_POINT('',(-0.339495522292874,-0.211524916601068,0.04));
#38019=CARTESIAN_POINT('Ctrl Pts',(-0.339495522292874,-0.211524916601068,
0.04));
#38020=CARTESIAN_POINT('Ctrl Pts',(-0.331889847003214,-0.199124959645674,
0.0269875185857514));
#38021=CARTESIAN_POINT('Ctrl Pts',(-0.324759526419164,-0.1875,0.0150000000000001));
#38022=CARTESIAN_POINT('',(-0.339495522292874,-0.211524916601068,0.245));
#38023=CARTESIAN_POINT('Origin',(-0.397137525113939,-0.18942488259565,0.5));
#38024=CARTESIAN_POINT('',(-0.352933712456347,-0.188249288476161,0.45));
#38025=CARTESIAN_POINT('Ctrl Pts',(-0.352933712456347,-0.188249288476161,
0.45));
#38026=CARTESIAN_POINT('Ctrl Pts',(-0.338392197082316,-0.187862558940078,
0.463012481414245));
#38027=CARTESIAN_POINT('Ctrl Pts',(-0.324759526419164,-0.1875,0.475));
#38028=CARTESIAN_POINT('',(-0.352933712456347,-0.188249288476161,0.04));
#38029=CARTESIAN_POINT('',(-0.352933712456347,-0.188249288476161,0.245));
#38030=CARTESIAN_POINT('Ctrl Pts',(-0.324759526419165,-0.1875,0.0150000000000001));
#38031=CARTESIAN_POINT('Ctrl Pts',(-0.338392197082305,-0.187862558940078,
0.0269875185857457));
#38032=CARTESIAN_POINT('Ctrl Pts',(-0.352933712456347,-0.188249288476161,
0.04));
#38033=CARTESIAN_POINT('Origin',(-0.375,4.59242549680257E-17,0.5));
#38034=CARTESIAN_POINT('',(-0.375,4.59242549680257E-17,0.475));
#38035=CARTESIAN_POINT('',(-0.399774205077229,-0.0134381901634729,0.45));
#38036=CARTESIAN_POINT('Ctrl Pts',(-0.375,4.59242549680257E-17,0.475));
#38037=CARTESIAN_POINT('Ctrl Pts',(-0.386987518585757,-0.00650235007910003,
0.463012481414244));
#38038=CARTESIAN_POINT('Ctrl Pts',(-0.399774205077229,-0.0134381901634728,
0.45));
#38039=CARTESIAN_POINT('',(-0.375,4.59242549680257E-17,0.015));
#38040=CARTESIAN_POINT('',(-0.375,4.59242549680257E-17,0.5));
#38041=CARTESIAN_POINT('',(-0.399774205077229,-0.0134381901634729,0.04));
#38042=CARTESIAN_POINT('Ctrl Pts',(-0.399774205077229,-0.0134381901634728,
0.04));
#38043=CARTESIAN_POINT('Ctrl Pts',(-0.386987518585752,-0.00650235007909753,
0.0269875185857518));
#38044=CARTESIAN_POINT('Ctrl Pts',(-0.375,4.59242549680257E-17,0.015));
#38045=CARTESIAN_POINT('',(-0.399774205077229,-0.0134381901634729,0.245));
#38046=CARTESIAN_POINT('Origin',(-0.438643626842576,0.0345220021202518,
0.5));
#38047=CARTESIAN_POINT('',(-0.399774205077229,0.013438190163473,0.45));
#38048=CARTESIAN_POINT('Ctrl Pts',(-0.399774205077229,0.013438190163473,
0.45));
#38049=CARTESIAN_POINT('Ctrl Pts',(-0.38698751858575,0.00650235007909647,
0.46301248141425));
#38050=CARTESIAN_POINT('Ctrl Pts',(-0.375,4.59242549680257E-17,0.475));
#38051=CARTESIAN_POINT('',(-0.399774205077229,0.013438190163473,0.04));
#38052=CARTESIAN_POINT('',(-0.399774205077229,0.013438190163473,0.245));
#38053=CARTESIAN_POINT('Ctrl Pts',(-0.375,4.59242549680257E-17,0.015));
#38054=CARTESIAN_POINT('Ctrl Pts',(-0.386987518585749,0.00650235007909624,
0.0269875185857492));
#38055=CARTESIAN_POINT('Ctrl Pts',(-0.399774205077229,0.013438190163473,
0.04));
#38056=CARTESIAN_POINT('Origin',(-0.362222184858401,0.0970571419134454,
0.5));
#38057=CARTESIAN_POINT('',(-0.362222184858401,0.0970571419134454,0.475));
#38058=CARTESIAN_POINT('',(-0.389630288914294,0.0904888830772256,0.45));
#38059=CARTESIAN_POINT('Ctrl Pts',(-0.362222184858401,0.0970571419134454,
0.475));
#38060=CARTESIAN_POINT('Ctrl Pts',(-0.375484170691896,0.0938789521539844,
0.463012481414245));
#38061=CARTESIAN_POINT('Ctrl Pts',(-0.389630288914294,0.0904888830772256,
0.45));
#38062=CARTESIAN_POINT('',(-0.362222184858401,0.0970571419134454,0.015));
#38063=CARTESIAN_POINT('',(-0.362222184858401,0.0970571419134454,0.5));
#38064=CARTESIAN_POINT('',(-0.389630288914294,0.0904888830772256,0.04));
#38065=CARTESIAN_POINT('Ctrl Pts',(-0.389630288914294,0.0904888830772256,
0.04));
#38066=CARTESIAN_POINT('Ctrl Pts',(-0.375484170691898,0.093878952153984,
0.0269875185857566));
#38067=CARTESIAN_POINT('Ctrl Pts',(-0.362222184858401,0.0970571419134454,
0.015));
#38068=CARTESIAN_POINT('',(-0.389630288914294,0.0904888830772256,0.245));
#38069=CARTESIAN_POINT('Origin',(-0.414762256080559,0.146875018062859,0.5));
#38070=CARTESIAN_POINT('',(-0.382674169822262,0.11644947295219,0.45));
#38071=CARTESIAN_POINT('Ctrl Pts',(-0.382674169822262,0.11644947295219,
0.45));
#38072=CARTESIAN_POINT('Ctrl Pts',(-0.372118306615107,0.106440527899934,
0.463012481414244));
#38073=CARTESIAN_POINT('Ctrl Pts',(-0.362222184858401,0.0970571419134454,
0.475));
#38074=CARTESIAN_POINT('',(-0.382674169822262,0.11644947295219,0.04));
#38075=CARTESIAN_POINT('',(-0.382674169822262,0.11644947295219,0.245));
#38076=CARTESIAN_POINT('Ctrl Pts',(-0.362222184858401,0.0970571419134454,
0.015));
#38077=CARTESIAN_POINT('Ctrl Pts',(-0.372118306615099,0.106440527899927,
0.026987518585746));
#38078=CARTESIAN_POINT('Ctrl Pts',(-0.382674169822262,0.11644947295219,
0.04));
#38079=CARTESIAN_POINT('Origin',(-0.265165042944955,0.265165042944955,0.5));
#38080=CARTESIAN_POINT('',(-0.265165042944955,0.265165042944955,0.475));
#38081=CARTESIAN_POINT('',(-0.292185286745036,0.273180815962104,0.45));
#38082=CARTESIAN_POINT('Ctrl Pts',(-0.265165042944955,0.265165042944955,
0.475));
#38083=CARTESIAN_POINT('Ctrl Pts',(-0.278239354461118,0.269043642791961,
0.463012481414249));
#38084=CARTESIAN_POINT('Ctrl Pts',(-0.292185286745036,0.273180815962104,
0.45));
#38085=CARTESIAN_POINT('',(-0.265165042944955,0.265165042944955,0.015));
#38086=CARTESIAN_POINT('',(-0.265165042944955,0.265165042944955,0.5));
#38087=CARTESIAN_POINT('',(-0.292185286745036,0.273180815962104,0.04));
#38088=CARTESIAN_POINT('Ctrl Pts',(-0.292185286745036,0.273180815962104,
0.04));
#38089=CARTESIAN_POINT('Ctrl Pts',(-0.278239354461119,0.269043642791962,
0.026987518585752));
#38090=CARTESIAN_POINT('Ctrl Pts',(-0.265165042944955,0.265165042944955,
0.015));
#38091=CARTESIAN_POINT('',(-0.292185286745036,0.273180815962104,0.245));
#38092=CARTESIAN_POINT('Origin',(-0.285757141265281,0.334578624864014,0.5));
#38093=CARTESIAN_POINT('',(-0.273180815962104,0.292185286745036,0.45));
#38094=CARTESIAN_POINT('Ctrl Pts',(-0.273180815962104,0.292185286745036,
0.45));
#38095=CARTESIAN_POINT('Ctrl Pts',(-0.26904364279196,0.278239354461116,
0.463012481414251));
#38096=CARTESIAN_POINT('Ctrl Pts',(-0.265165042944955,0.265165042944955,
0.475));
#38097=CARTESIAN_POINT('',(-0.273180815962104,0.292185286745036,0.04));
#38098=CARTESIAN_POINT('',(-0.273180815962104,0.292185286745036,0.245));
#38099=CARTESIAN_POINT('Ctrl Pts',(-0.265165042944955,0.265165042944955,
0.015));
#38100=CARTESIAN_POINT('Ctrl Pts',(-0.269043642791957,0.278239354461105,
0.0269875185857388));
#38101=CARTESIAN_POINT('Ctrl Pts',(-0.273180815962104,0.292185286745036,
0.04));
#38102=CARTESIAN_POINT('Origin',(-0.0970571419134453,0.362222184858401,
0.5));
#38103=CARTESIAN_POINT('',(-0.0970571419134453,0.362222184858401,0.475));
#38104=CARTESIAN_POINT('',(-0.11644947295219,0.382674169822262,0.45));
#38105=CARTESIAN_POINT('Ctrl Pts',(-0.0970571419134453,0.362222184858401,
0.475));
#38106=CARTESIAN_POINT('Ctrl Pts',(-0.106440527899932,0.372118306615104,
0.463012481414248));
#38107=CARTESIAN_POINT('Ctrl Pts',(-0.11644947295219,0.382674169822262,
0.45));
#38108=CARTESIAN_POINT('',(-0.0970571419134453,0.362222184858401,0.015));
#38109=CARTESIAN_POINT('',(-0.0970571419134453,0.362222184858401,0.5));
#38110=CARTESIAN_POINT('',(-0.11644947295219,0.382674169822262,0.04));
#38111=CARTESIAN_POINT('Ctrl Pts',(-0.11644947295219,0.382674169822262,
0.04));
#38112=CARTESIAN_POINT('Ctrl Pts',(-0.106440527899929,0.372118306615102,
0.0269875185857486));
#38113=CARTESIAN_POINT('Ctrl Pts',(-0.0970571419134453,0.362222184858401,
0.015));
#38114=CARTESIAN_POINT('',(-0.11644947295219,0.382674169822262,0.245));
#38115=CARTESIAN_POINT('Origin',(-0.0801836312165449,0.43263215932814,0.5));
#38116=CARTESIAN_POINT('',(-0.0904888830772255,0.389630288914294,0.45));
#38117=CARTESIAN_POINT('Ctrl Pts',(-0.0904888830772256,0.389630288914294,
0.45));
#38118=CARTESIAN_POINT('Ctrl Pts',(-0.0938789521539861,0.375484170691889,
0.463012481414251));
#38119=CARTESIAN_POINT('Ctrl Pts',(-0.0970571419134453,0.362222184858401,
0.475));
#38120=CARTESIAN_POINT('',(-0.0904888830772255,0.389630288914294,0.04));
#38121=CARTESIAN_POINT('',(-0.0904888830772255,0.389630288914294,0.245));
#38122=CARTESIAN_POINT('Ctrl Pts',(-0.0970571419134453,0.362222184858401,
0.015));
#38123=CARTESIAN_POINT('Ctrl Pts',(-0.093878952153988,0.375484170691881,
0.0269875185857416));
#38124=CARTESIAN_POINT('Ctrl Pts',(-0.0904888830772256,0.389630288914294,
0.04));
#38125=CARTESIAN_POINT('Origin',(0.0970571419134453,0.362222184858401,0.5));
#38126=CARTESIAN_POINT('',(0.0970571419134453,0.362222184858401,0.475));
#38127=CARTESIAN_POINT('',(0.0904888830772255,0.389630288914294,0.45));
#38128=CARTESIAN_POINT('Ctrl Pts',(0.0970571419134453,0.362222184858401,
0.475));
#38129=CARTESIAN_POINT('Ctrl Pts',(0.093878952153984,0.375484170691898,
0.463012481414244));
#38130=CARTESIAN_POINT('Ctrl Pts',(0.0904888830772255,0.389630288914294,
0.45));
#38131=CARTESIAN_POINT('',(0.0970571419134453,0.362222184858401,0.015));
#38132=CARTESIAN_POINT('',(0.0970571419134453,0.362222184858401,0.5));
#38133=CARTESIAN_POINT('',(0.0904888830772255,0.389630288914294,0.04));
#38134=CARTESIAN_POINT('Ctrl Pts',(0.0904888830772255,0.389630288914294,
0.04));
#38135=CARTESIAN_POINT('Ctrl Pts',(0.0938789521539869,0.375484170691886,
0.0269875185857455));
#38136=CARTESIAN_POINT('Ctrl Pts',(0.0970571419134453,0.362222184858401,
0.015));
#38137=CARTESIAN_POINT('',(0.0904888830772255,0.389630288914294,0.245));
#38138=CARTESIAN_POINT('Origin',(0.146875018062859,0.414762256080559,0.5));
#38139=CARTESIAN_POINT('',(0.11644947295219,0.382674169822262,0.45));
#38140=CARTESIAN_POINT('Ctrl Pts',(0.11644947295219,0.382674169822262,0.45));
#38141=CARTESIAN_POINT('Ctrl Pts',(0.106440527899934,0.372118306615107,
0.463012481414245));
#38142=CARTESIAN_POINT('Ctrl Pts',(0.0970571419134453,0.362222184858401,
0.475));
#38143=CARTESIAN_POINT('',(0.11644947295219,0.382674169822262,0.04));
#38144=CARTESIAN_POINT('',(0.11644947295219,0.382674169822262,0.245));
#38145=CARTESIAN_POINT('Ctrl Pts',(0.0970571419134453,0.362222184858401,
0.015));
#38146=CARTESIAN_POINT('Ctrl Pts',(0.106440527899938,0.372118306615111,
0.0269875185857598));
#38147=CARTESIAN_POINT('Ctrl Pts',(0.11644947295219,0.382674169822262,0.04));
#38148=CARTESIAN_POINT('Origin',(0.265165042944955,0.265165042944955,0.5));
#38149=CARTESIAN_POINT('',(0.265165042944955,0.265165042944955,0.475));
#38150=CARTESIAN_POINT('',(0.273180815962104,0.292185286745036,0.45));
#38151=CARTESIAN_POINT('Ctrl Pts',(0.265165042944955,0.265165042944955,
0.475));
#38152=CARTESIAN_POINT('Ctrl Pts',(0.269043642791962,0.27823935446112,0.463012481414247));
#38153=CARTESIAN_POINT('Ctrl Pts',(0.273180815962104,0.292185286745036,
0.45));
#38154=CARTESIAN_POINT('',(0.265165042944955,0.265165042944955,0.015));
#38155=CARTESIAN_POINT('',(0.265165042944955,0.265165042944955,0.5));
#38156=CARTESIAN_POINT('',(0.273180815962104,0.292185286745036,0.04));
#38157=CARTESIAN_POINT('Ctrl Pts',(0.273180815962104,0.292185286745036,
0.04));
#38158=CARTESIAN_POINT('Ctrl Pts',(0.26904364279196,0.278239354461114,0.0269875185857475));
#38159=CARTESIAN_POINT('Ctrl Pts',(0.265165042944955,0.265165042944955,
0.015));
#38160=CARTESIAN_POINT('',(0.273180815962104,0.292185286745036,0.245));
#38161=CARTESIAN_POINT('Origin',(0.334578624864014,0.285757141265281,0.5));
#38162=CARTESIAN_POINT('',(0.292185286745036,0.273180815962104,0.45));
#38163=CARTESIAN_POINT('Ctrl Pts',(0.292185286745036,0.273180815962104,
0.45));
#38164=CARTESIAN_POINT('Ctrl Pts',(0.278239354461118,0.269043642791961,
0.463012481414249));
#38165=CARTESIAN_POINT('Ctrl Pts',(0.265165042944955,0.265165042944955,
0.475));
#38166=CARTESIAN_POINT('',(0.292185286745036,0.273180815962104,0.04));
#38167=CARTESIAN_POINT('',(0.292185286745036,0.273180815962104,0.245));
#38168=CARTESIAN_POINT('Ctrl Pts',(0.265165042944955,0.265165042944955,
0.015));
#38169=CARTESIAN_POINT('Ctrl Pts',(0.278239354461114,0.26904364279196,0.0269875185857475));
#38170=CARTESIAN_POINT('Ctrl Pts',(0.292185286745036,0.273180815962104,
0.04));
#38171=CARTESIAN_POINT('Origin',(0.362222184858401,0.0970571419134453,0.5));
#38172=CARTESIAN_POINT('',(0.362222184858401,0.0970571419134453,0.475));
#38173=CARTESIAN_POINT('',(0.382674169822262,0.11644947295219,0.45));
#38174=CARTESIAN_POINT('Ctrl Pts',(0.362222184858401,0.0970571419134453,
0.475));
#38175=CARTESIAN_POINT('Ctrl Pts',(0.372118306615106,0.106440527899933,
0.463012481414246));
#38176=CARTESIAN_POINT('Ctrl Pts',(0.382674169822262,0.11644947295219,0.45));
#38177=CARTESIAN_POINT('',(0.362222184858401,0.0970571419134453,0.015));
#38178=CARTESIAN_POINT('',(0.362222184858401,0.0970571419134453,0.5));
#38179=CARTESIAN_POINT('',(0.382674169822262,0.11644947295219,0.04));
#38180=CARTESIAN_POINT('Ctrl Pts',(0.382674169822262,0.11644947295219,0.04));
#38181=CARTESIAN_POINT('Ctrl Pts',(0.372118306615112,0.106440527899938,
0.0269875185857607));
#38182=CARTESIAN_POINT('Ctrl Pts',(0.362222184858401,0.0970571419134453,
0.015));
#38183=CARTESIAN_POINT('',(0.382674169822262,0.11644947295219,0.245));
#38184=CARTESIAN_POINT('Origin',(0.43263215932814,0.0801836312165449,0.5));
#38185=CARTESIAN_POINT('',(0.389630288914294,0.0904888830772255,0.45));
#38186=CARTESIAN_POINT('Ctrl Pts',(0.389630288914294,0.0904888830772255,
0.45));
#38187=CARTESIAN_POINT('Ctrl Pts',(0.375484170691896,0.0938789521539845,
0.463012481414246));
#38188=CARTESIAN_POINT('Ctrl Pts',(0.362222184858401,0.0970571419134453,
0.475));
#38189=CARTESIAN_POINT('',(0.389630288914294,0.0904888830772255,0.04));
#38190=CARTESIAN_POINT('',(0.389630288914294,0.0904888830772255,0.245));
#38191=CARTESIAN_POINT('Ctrl Pts',(0.362222184858401,0.0970571419134453,
0.015));
#38192=CARTESIAN_POINT('Ctrl Pts',(0.375484170691883,0.0938789521539875,
0.0269875185857432));
#38193=CARTESIAN_POINT('Ctrl Pts',(0.389630288914294,0.0904888830772255,
0.04));
#38194=CARTESIAN_POINT('Origin',(0.324759526419165,0.1875,0.5));
#38195=CARTESIAN_POINT('',(0.324759526419165,0.1875,0.475));
#38196=CARTESIAN_POINT('',(0.339495522292874,0.211524916601068,0.45));
#38197=CARTESIAN_POINT('Ctrl Pts',(0.324759526419165,0.1875,0.475));
#38198=CARTESIAN_POINT('Ctrl Pts',(0.331889847003213,0.199124959645671,
0.463012481414251));
#38199=CARTESIAN_POINT('Ctrl Pts',(0.339495522292874,0.211524916601068,
0.45));
#38200=CARTESIAN_POINT('',(0.324759526419165,0.1875,0.015));
#38201=CARTESIAN_POINT('',(0.324759526419165,0.1875,0.5));
#38202=CARTESIAN_POINT('',(0.339495522292874,0.211524916601068,0.04));
#38203=CARTESIAN_POINT('Ctrl Pts',(0.339495522292874,0.211524916601068,
0.04));
#38204=CARTESIAN_POINT('Ctrl Pts',(0.331889847003218,0.199124959645679,
0.0269875185857566));
#38205=CARTESIAN_POINT('Ctrl Pts',(0.324759526419165,0.1875,0.015));
#38206=CARTESIAN_POINT('',(0.339495522292874,0.211524916601068,0.245));
#38207=CARTESIAN_POINT('Origin',(0.397137525113939,0.18942488259565,0.5));
#38208=CARTESIAN_POINT('',(0.352933712456347,0.188249288476161,0.45));
#38209=CARTESIAN_POINT('Ctrl Pts',(0.352933712456347,0.188249288476161,
0.45));
#38210=CARTESIAN_POINT('Ctrl Pts',(0.338392197082318,0.187862558940078,
0.463012481414243));
#38211=CARTESIAN_POINT('Ctrl Pts',(0.324759526419165,0.1875,0.475));
#38212=CARTESIAN_POINT('',(0.352933712456347,0.188249288476161,0.04));
#38213=CARTESIAN_POINT('',(0.352933712456347,0.188249288476161,0.245));
#38214=CARTESIAN_POINT('Ctrl Pts',(0.324759526419165,0.1875,0.015));
#38215=CARTESIAN_POINT('Ctrl Pts',(0.338392197082309,0.187862558940078,
0.0269875185857488));
#38216=CARTESIAN_POINT('Ctrl Pts',(0.352933712456347,0.188249288476161,
0.04));
#38217=CARTESIAN_POINT('Origin',(0.1875,0.324759526419164,0.5));
#38218=CARTESIAN_POINT('',(0.1875,0.324759526419164,0.475));
#38219=CARTESIAN_POINT('',(0.188249288476161,0.352933712456347,0.45));
#38220=CARTESIAN_POINT('Ctrl Pts',(0.1875,0.324759526419164,0.475));
#38221=CARTESIAN_POINT('Ctrl Pts',(0.187862558940078,0.338392197082313,
0.463012481414248));
#38222=CARTESIAN_POINT('Ctrl Pts',(0.188249288476161,0.352933712456347,
0.45));
#38223=CARTESIAN_POINT('',(0.1875,0.324759526419164,0.0150000000000001));
#38224=CARTESIAN_POINT('',(0.1875,0.324759526419164,0.5));
#38225=CARTESIAN_POINT('',(0.188249288476161,0.352933712456347,0.04));
#38226=CARTESIAN_POINT('Ctrl Pts',(0.188249288476161,0.352933712456347,
0.04));
#38227=CARTESIAN_POINT('Ctrl Pts',(0.187862558940078,0.338392197082318,
0.0269875185857566));
#38228=CARTESIAN_POINT('Ctrl Pts',(0.1875,0.324759526419164,0.0150000000000001));
#38229=CARTESIAN_POINT('',(0.188249288476161,0.352933712456347,0.245));
#38230=CARTESIAN_POINT('Origin',(0.249218744246926,0.362615522993687,0.5));
#38231=CARTESIAN_POINT('',(0.211524916601068,0.339495522292874,0.45));
#38232=CARTESIAN_POINT('Ctrl Pts',(0.211524916601068,0.339495522292874,
0.45));
#38233=CARTESIAN_POINT('Ctrl Pts',(0.199124959645677,0.331889847003217,
0.463012481414245));
#38234=CARTESIAN_POINT('Ctrl Pts',(0.1875,0.324759526419164,0.475));
#38235=CARTESIAN_POINT('',(0.211524916601068,0.339495522292874,0.04));
#38236=CARTESIAN_POINT('',(0.211524916601068,0.339495522292874,0.245));
#38237=CARTESIAN_POINT('Ctrl Pts',(0.1875,0.324759526419164,0.015));
#38238=CARTESIAN_POINT('Ctrl Pts',(0.199124959645668,0.331889847003211,
0.0269875185857458));
#38239=CARTESIAN_POINT('Ctrl Pts',(0.211524916601068,0.339495522292874,
0.04));
#38240=CARTESIAN_POINT('Origin',(2.29621274840129E-17,0.375,0.5));
#38241=CARTESIAN_POINT('',(2.29621274840129E-17,0.375,0.475));
#38242=CARTESIAN_POINT('',(-0.0134381901634729,0.399774205077229,0.45));
#38243=CARTESIAN_POINT('Ctrl Pts',(2.29621274840129E-17,0.375,0.475));
#38244=CARTESIAN_POINT('Ctrl Pts',(-0.00650235007909964,0.386987518585756,
0.463012481414244));
#38245=CARTESIAN_POINT('Ctrl Pts',(-0.0134381901634728,0.399774205077229,
0.45));
#38246=CARTESIAN_POINT('',(2.29621274840129E-17,0.375,0.015));
#38247=CARTESIAN_POINT('',(2.29621274840129E-17,0.375,0.5));
#38248=CARTESIAN_POINT('',(-0.0134381901634729,0.399774205077229,0.04));
#38249=CARTESIAN_POINT('Ctrl Pts',(-0.0134381901634729,0.399774205077229,
0.04));
#38250=CARTESIAN_POINT('Ctrl Pts',(-0.00650235007909639,0.38698751858575,
0.0269875185857497));
#38251=CARTESIAN_POINT('Ctrl Pts',(2.29621274840129E-17,0.375,0.015));
#38252=CARTESIAN_POINT('',(-0.0134381901634729,0.399774205077229,0.245));
#38253=CARTESIAN_POINT('Origin',(0.0345220021202518,0.438643626842576,0.5));
#38254=CARTESIAN_POINT('',(0.013438190163473,0.399774205077229,0.45));
#38255=CARTESIAN_POINT('Ctrl Pts',(0.013438190163473,0.399774205077229,
0.45));
#38256=CARTESIAN_POINT('Ctrl Pts',(0.00650235007909615,0.386987518585749,
0.463012481414251));
#38257=CARTESIAN_POINT('Ctrl Pts',(2.29621274840129E-17,0.375,0.475));
#38258=CARTESIAN_POINT('',(0.013438190163473,0.399774205077229,0.04));
#38259=CARTESIAN_POINT('',(0.013438190163473,0.399774205077229,0.245));
#38260=CARTESIAN_POINT('Ctrl Pts',(2.29621274840129E-17,0.375,0.015));
#38261=CARTESIAN_POINT('Ctrl Pts',(0.00650235007909749,0.386987518585752,
0.0269875185857516));
#38262=CARTESIAN_POINT('Ctrl Pts',(0.013438190163473,0.399774205077229,
0.04));
#38263=CARTESIAN_POINT('Origin',(-0.1875,0.324759526419165,0.5));
#38264=CARTESIAN_POINT('',(-0.1875,0.324759526419165,0.475));
#38265=CARTESIAN_POINT('',(-0.211524916601068,0.339495522292874,0.45));
#38266=CARTESIAN_POINT('Ctrl Pts',(-0.1875,0.324759526419165,0.475));
#38267=CARTESIAN_POINT('Ctrl Pts',(-0.199124959645671,0.331889847003213,
0.463012481414252));
#38268=CARTESIAN_POINT('Ctrl Pts',(-0.211524916601068,0.339495522292874,
0.45));
#38269=CARTESIAN_POINT('',(-0.1875,0.324759526419165,0.015));
#38270=CARTESIAN_POINT('',(-0.1875,0.324759526419165,0.5));
#38271=CARTESIAN_POINT('',(-0.211524916601068,0.339495522292874,0.04));
#38272=CARTESIAN_POINT('Ctrl Pts',(-0.211524916601068,0.339495522292874,
0.04));
#38273=CARTESIAN_POINT('Ctrl Pts',(-0.199124959645683,0.33188984700322,
0.0269875185857606));
#38274=CARTESIAN_POINT('Ctrl Pts',(-0.1875,0.324759526419165,0.015));
#38275=CARTESIAN_POINT('',(-0.211524916601068,0.339495522292874,0.245));
#38276=CARTESIAN_POINT('Origin',(-0.18942488259565,0.397137525113939,0.5));
#38277=CARTESIAN_POINT('',(-0.188249288476161,0.352933712456347,0.45));
#38278=CARTESIAN_POINT('Ctrl Pts',(-0.188249288476161,0.352933712456347,
0.45));
#38279=CARTESIAN_POINT('Ctrl Pts',(-0.187862558940078,0.33839219708231,
0.46301248141425));
#38280=CARTESIAN_POINT('Ctrl Pts',(-0.1875,0.324759526419165,0.475));
#38281=CARTESIAN_POINT('',(-0.188249288476161,0.352933712456347,0.04));
#38282=CARTESIAN_POINT('',(-0.188249288476161,0.352933712456347,0.245));
#38283=CARTESIAN_POINT('Ctrl Pts',(-0.1875,0.324759526419165,0.015));
#38284=CARTESIAN_POINT('Ctrl Pts',(-0.187862558940077,0.338392197082308,
0.0269875185857478));
#38285=CARTESIAN_POINT('Ctrl Pts',(-0.188249288476161,0.352933712456347,
0.04));
#38286=CARTESIAN_POINT('Origin',(-0.324759526419165,0.1875,0.5));
#38287=CARTESIAN_POINT('',(-0.324759526419165,0.1875,0.475));
#38288=CARTESIAN_POINT('',(-0.352933712456347,0.188249288476161,0.45));
#38289=CARTESIAN_POINT('Ctrl Pts',(-0.324759526419165,0.1875,0.475));
#38290=CARTESIAN_POINT('Ctrl Pts',(-0.338392197082309,0.187862558940077,
0.463012481414251));
#38291=CARTESIAN_POINT('Ctrl Pts',(-0.352933712456347,0.188249288476161,
0.45));
#38292=CARTESIAN_POINT('',(-0.324759526419165,0.1875,0.015));
#38293=CARTESIAN_POINT('',(-0.324759526419165,0.1875,0.5));
#38294=CARTESIAN_POINT('',(-0.352933712456347,0.188249288476161,0.04));
#38295=CARTESIAN_POINT('Ctrl Pts',(-0.352933712456347,0.188249288476161,
0.04));
#38296=CARTESIAN_POINT('Ctrl Pts',(-0.338392197082316,0.187862558940078,
0.0269875185857554));
#38297=CARTESIAN_POINT('Ctrl Pts',(-0.324759526419165,0.1875,0.015));
#38298=CARTESIAN_POINT('',(-0.352933712456347,0.188249288476161,0.245));
#38299=CARTESIAN_POINT('Origin',(-0.362615522993687,0.249218744246926,0.5));
#38300=CARTESIAN_POINT('',(-0.339495522292874,0.211524916601068,0.45));
#38301=CARTESIAN_POINT('Ctrl Pts',(-0.339495522292874,0.211524916601068,
0.45));
#38302=CARTESIAN_POINT('Ctrl Pts',(-0.331889847003215,0.199124959645674,
0.463012481414249));
#38303=CARTESIAN_POINT('Ctrl Pts',(-0.324759526419165,0.1875,0.475));
#38304=CARTESIAN_POINT('',(-0.339495522292874,0.211524916601068,0.04));
#38305=CARTESIAN_POINT('',(-0.339495522292874,0.211524916601068,0.245));
#38306=CARTESIAN_POINT('Ctrl Pts',(-0.324759526419164,0.1875,0.015));
#38307=CARTESIAN_POINT('Ctrl Pts',(-0.331889847003215,0.199124959645674,
0.0269875185857514));
#38308=CARTESIAN_POINT('Ctrl Pts',(-0.339495522292874,0.211524916601068,
0.04));
#38309=CARTESIAN_POINT('Origin',(0.375,0.,0.5));
#38310=CARTESIAN_POINT('',(0.375,0.,0.475));
#38311=CARTESIAN_POINT('',(0.399774205077229,0.013438190163473,0.45));
#38312=CARTESIAN_POINT('Ctrl Pts',(0.375,0.,0.475));
#38313=CARTESIAN_POINT('Ctrl Pts',(0.386987518585754,0.00650235007909865,
0.463012481414246));
#38314=CARTESIAN_POINT('Ctrl Pts',(0.399774205077229,0.0134381901634729,
0.45));
#38315=CARTESIAN_POINT('',(0.375,0.,0.015));
#38316=CARTESIAN_POINT('',(0.375,0.,0.5));
#38317=CARTESIAN_POINT('',(0.399774205077229,0.013438190163473,0.04));
#38318=CARTESIAN_POINT('Ctrl Pts',(0.399774205077229,0.0134381901634729,
0.04));
#38319=CARTESIAN_POINT('Ctrl Pts',(0.38698751858575,0.00650235007909652,
0.02698751858575));
#38320=CARTESIAN_POINT('Ctrl Pts',(0.375,0.,0.015));
#38321=CARTESIAN_POINT('',(0.399774205077229,0.013438190163473,0.245));
#38322=CARTESIAN_POINT('Origin',(0.438643626842576,-0.0345220021202518,
0.5));
#38323=CARTESIAN_POINT('',(0.399774205077229,-0.013438190163473,0.45));
#38324=CARTESIAN_POINT('Ctrl Pts',(0.399774205077229,-0.0134381901634729,
0.45));
#38325=CARTESIAN_POINT('Ctrl Pts',(0.386987518585751,-0.00650235007909692,
0.463012481414249));
#38326=CARTESIAN_POINT('Ctrl Pts',(0.375,0.,0.475));
#38327=CARTESIAN_POINT('',(0.399774205077229,-0.013438190163473,0.04));
#38328=CARTESIAN_POINT('',(0.399774205077229,-0.013438190163473,0.245));
#38329=CARTESIAN_POINT('Ctrl Pts',(0.375,0.,0.015));
#38330=CARTESIAN_POINT('Ctrl Pts',(0.386987518585746,-0.00650235007909417,
0.0269875185857456));
#38331=CARTESIAN_POINT('Ctrl Pts',(0.399774205077229,-0.0134381901634729,
0.04));
#38332=CARTESIAN_POINT('Origin',(-0.362222184858401,-0.0970571419134453,
0.5));
#38333=CARTESIAN_POINT('',(-0.362222184858401,-0.0970571419134453,0.475));
#38334=CARTESIAN_POINT('',(-0.382674169822262,-0.11644947295219,0.45));
#38335=CARTESIAN_POINT('Ctrl Pts',(-0.362222184858401,-0.0970571419134453,
0.475));
#38336=CARTESIAN_POINT('Ctrl Pts',(-0.372118306615105,-0.106440527899932,
0.463012481414247));
#38337=CARTESIAN_POINT('Ctrl Pts',(-0.382674169822262,-0.11644947295219,
0.45));
#38338=CARTESIAN_POINT('',(-0.362222184858401,-0.0970571419134453,0.015));
#38339=CARTESIAN_POINT('',(-0.362222184858401,-0.0970571419134453,0.5));
#38340=CARTESIAN_POINT('',(-0.382674169822262,-0.11644947295219,0.04));
#38341=CARTESIAN_POINT('Ctrl Pts',(-0.382674169822262,-0.11644947295219,
0.04));
#38342=CARTESIAN_POINT('Ctrl Pts',(-0.372118306615101,-0.106440527899928,
0.0269875185857478));
#38343=CARTESIAN_POINT('Ctrl Pts',(-0.362222184858401,-0.0970571419134453,
0.015));
#38344=CARTESIAN_POINT('',(-0.382674169822262,-0.11644947295219,0.245));
#38345=CARTESIAN_POINT('Origin',(-0.43263215932814,-0.0801836312165449,
0.5));
#38346=CARTESIAN_POINT('',(-0.389630288914294,-0.0904888830772255,0.45));
#38347=CARTESIAN_POINT('Ctrl Pts',(-0.389630288914294,-0.0904888830772256,
0.45));
#38348=CARTESIAN_POINT('Ctrl Pts',(-0.375484170691889,-0.093878952153986,
0.463012481414251));
#38349=CARTESIAN_POINT('Ctrl Pts',(-0.362222184858401,-0.0970571419134453,
0.475));
#38350=CARTESIAN_POINT('',(-0.389630288914294,-0.0904888830772255,0.04));
#38351=CARTESIAN_POINT('',(-0.389630288914294,-0.0904888830772255,0.245));
#38352=CARTESIAN_POINT('Ctrl Pts',(-0.362222184858401,-0.0970571419134453,
0.015));
#38353=CARTESIAN_POINT('Ctrl Pts',(-0.375484170691881,-0.0938789521539879,
0.0269875185857416));
#38354=CARTESIAN_POINT('Ctrl Pts',(-0.389630288914294,-0.0904888830772256,
0.04));
#38355=CARTESIAN_POINT('Origin',(-0.265165042944955,-0.265165042944955,
0.5));
#38356=CARTESIAN_POINT('',(-0.265165042944955,-0.265165042944955,0.475));
#38357=CARTESIAN_POINT('',(-0.273180815962104,-0.292185286745036,0.45));
#38358=CARTESIAN_POINT('Ctrl Pts',(-0.265165042944955,-0.265165042944955,
0.475));
#38359=CARTESIAN_POINT('Ctrl Pts',(-0.269043642791962,-0.278239354461122,
0.463012481414245));
#38360=CARTESIAN_POINT('Ctrl Pts',(-0.273180815962104,-0.292185286745036,
0.45));
#38361=CARTESIAN_POINT('',(-0.265165042944955,-0.265165042944955,0.015));
#38362=CARTESIAN_POINT('',(-0.265165042944955,-0.265165042944955,0.5));
#38363=CARTESIAN_POINT('',(-0.273180815962104,-0.292185286745036,0.04));
#38364=CARTESIAN_POINT('Ctrl Pts',(-0.273180815962104,-0.292185286745036,
0.04));
#38365=CARTESIAN_POINT('Ctrl Pts',(-0.269043642791963,-0.278239354461123,
0.0269875185857556));
#38366=CARTESIAN_POINT('Ctrl Pts',(-0.265165042944955,-0.265165042944955,
0.015));
#38367=CARTESIAN_POINT('',(-0.273180815962104,-0.292185286745036,0.245));
#38368=CARTESIAN_POINT('Origin',(-0.334578624864014,-0.285757141265281,
0.5));
#38369=CARTESIAN_POINT('',(-0.292185286745036,-0.273180815962104,0.45));
#38370=CARTESIAN_POINT('Ctrl Pts',(-0.292185286745036,-0.273180815962104,
0.45));
#38371=CARTESIAN_POINT('Ctrl Pts',(-0.278239354461122,-0.269043642791962,
0.463012481414245));
#38372=CARTESIAN_POINT('Ctrl Pts',(-0.265165042944955,-0.265165042944955,
0.475));
#38373=CARTESIAN_POINT('',(-0.292185286745036,-0.273180815962104,0.04));
#38374=CARTESIAN_POINT('',(-0.292185286745036,-0.273180815962104,0.245));
#38375=CARTESIAN_POINT('Ctrl Pts',(-0.265165042944955,-0.265165042944955,
0.015));
#38376=CARTESIAN_POINT('Ctrl Pts',(-0.278239354461126,-0.269043642791964,
0.0269875185857586));
#38377=CARTESIAN_POINT('Ctrl Pts',(-0.292185286745036,-0.273180815962104,
0.04));
#38378=CARTESIAN_POINT('Origin',(-0.0970571419134452,-0.362222184858401,
0.5));
#38379=CARTESIAN_POINT('',(-0.0970571419134452,-0.362222184858401,0.475));
#38380=CARTESIAN_POINT('',(-0.0904888830772255,-0.389630288914294,0.45));
#38381=CARTESIAN_POINT('Ctrl Pts',(-0.0970571419134452,-0.362222184858401,
0.475));
#38382=CARTESIAN_POINT('Ctrl Pts',(-0.0938789521539842,-0.375484170691897,
0.463012481414244));
#38383=CARTESIAN_POINT('Ctrl Pts',(-0.0904888830772255,-0.389630288914294,
0.45));
#38384=CARTESIAN_POINT('',(-0.0970571419134452,-0.362222184858401,0.015));
#38385=CARTESIAN_POINT('',(-0.0970571419134452,-0.362222184858401,0.5));
#38386=CARTESIAN_POINT('',(-0.0904888830772255,-0.389630288914294,0.04));
#38387=CARTESIAN_POINT('Ctrl Pts',(-0.0904888830772256,-0.389630288914294,
0.04));
#38388=CARTESIAN_POINT('Ctrl Pts',(-0.0938789521539856,-0.375484170691891,
0.0269875185857502));
#38389=CARTESIAN_POINT('Ctrl Pts',(-0.0970571419134452,-0.362222184858401,
0.015));
#38390=CARTESIAN_POINT('',(-0.0904888830772255,-0.389630288914294,0.245));
#38391=CARTESIAN_POINT('Origin',(-0.146875018062859,-0.414762256080559,
0.5));
#38392=CARTESIAN_POINT('',(-0.11644947295219,-0.382674169822262,0.45));
#38393=CARTESIAN_POINT('Ctrl Pts',(-0.11644947295219,-0.382674169822262,
0.45));
#38394=CARTESIAN_POINT('Ctrl Pts',(-0.106440527899936,-0.372118306615109,
0.463012481414242));
#38395=CARTESIAN_POINT('Ctrl Pts',(-0.0970571419134452,-0.362222184858401,
0.475));
#38396=CARTESIAN_POINT('',(-0.11644947295219,-0.382674169822262,0.04));
#38397=CARTESIAN_POINT('',(-0.11644947295219,-0.382674169822262,0.245));
#38398=CARTESIAN_POINT('Ctrl Pts',(-0.0970571419134452,-0.362222184858401,
0.015));
#38399=CARTESIAN_POINT('Ctrl Pts',(-0.106440527899943,-0.372118306615116,
0.0269875185857666));
#38400=CARTESIAN_POINT('Ctrl Pts',(-0.11644947295219,-0.382674169822262,
0.04));
#38401=CARTESIAN_POINT('Origin',(0.0970571419134451,-0.362222184858401,
0.5));
#38402=CARTESIAN_POINT('',(0.0970571419134451,-0.362222184858401,0.475));
#38403=CARTESIAN_POINT('',(0.11644947295219,-0.382674169822262,0.45));
#38404=CARTESIAN_POINT('Ctrl Pts',(0.0970571419134451,-0.362222184858401,
0.475));
#38405=CARTESIAN_POINT('Ctrl Pts',(0.106440527899935,-0.372118306615108,
0.463012481414243));
#38406=CARTESIAN_POINT('Ctrl Pts',(0.11644947295219,-0.382674169822262,
0.45));
#38407=CARTESIAN_POINT('',(0.0970571419134451,-0.362222184858401,0.0150000000000001));
#38408=CARTESIAN_POINT('',(0.0970571419134451,-0.362222184858401,0.5));
#38409=CARTESIAN_POINT('',(0.11644947295219,-0.382674169822262,0.04));
#38410=CARTESIAN_POINT('Ctrl Pts',(0.11644947295219,-0.382674169822262,
0.04));
#38411=CARTESIAN_POINT('Ctrl Pts',(0.106440527899933,-0.372118306615106,
0.0269875185857537));
#38412=CARTESIAN_POINT('Ctrl Pts',(0.0970571419134451,-0.362222184858401,
0.0150000000000001));
#38413=CARTESIAN_POINT('',(0.11644947295219,-0.382674169822262,0.245));
#38414=CARTESIAN_POINT('Origin',(0.0801836312165449,-0.43263215932814,0.5));
#38415=CARTESIAN_POINT('',(0.0904888830772254,-0.389630288914294,0.45));
#38416=CARTESIAN_POINT('Ctrl Pts',(0.0904888830772254,-0.389630288914294,
0.45));
#38417=CARTESIAN_POINT('Ctrl Pts',(0.0938789521539843,-0.375484170691896,
0.463012481414245));
#38418=CARTESIAN_POINT('Ctrl Pts',(0.0970571419134451,-0.362222184858401,
0.475));
#38419=CARTESIAN_POINT('',(0.0904888830772254,-0.389630288914294,0.04));
#38420=CARTESIAN_POINT('',(0.0904888830772254,-0.389630288914294,0.245));
#38421=CARTESIAN_POINT('Ctrl Pts',(0.0970571419134451,-0.362222184858401,
0.0150000000000001));
#38422=CARTESIAN_POINT('Ctrl Pts',(0.0938789521539861,-0.375484170691888,
0.0269875185857479));
#38423=CARTESIAN_POINT('Ctrl Pts',(0.0904888830772254,-0.389630288914294,
0.04));
#38424=CARTESIAN_POINT('Origin',(0.265165042944955,-0.265165042944955,0.5));
#38425=CARTESIAN_POINT('',(0.265165042944955,-0.265165042944955,0.475));
#38426=CARTESIAN_POINT('',(0.292185286745036,-0.273180815962104,0.45));
#38427=CARTESIAN_POINT('Ctrl Pts',(0.265165042944955,-0.265165042944955,
0.475));
#38428=CARTESIAN_POINT('Ctrl Pts',(0.278239354461118,-0.269043642791961,
0.463012481414249));
#38429=CARTESIAN_POINT('Ctrl Pts',(0.292185286745036,-0.273180815962104,
0.45));
#38430=CARTESIAN_POINT('',(0.265165042944955,-0.265165042944955,0.015));
#38431=CARTESIAN_POINT('',(0.265165042944955,-0.265165042944955,0.5));
#38432=CARTESIAN_POINT('',(0.292185286745036,-0.273180815962104,0.04));
#38433=CARTESIAN_POINT('Ctrl Pts',(0.292185286745036,-0.273180815962104,
0.04));
#38434=CARTESIAN_POINT('Ctrl Pts',(0.278239354461123,-0.269043642791963,
0.0269875185857557));
#38435=CARTESIAN_POINT('Ctrl Pts',(0.265165042944955,-0.265165042944955,
0.015));
#38436=CARTESIAN_POINT('',(0.292185286745036,-0.273180815962104,0.245));
#38437=CARTESIAN_POINT('Origin',(0.285757141265281,-0.334578624864014,0.5));
#38438=CARTESIAN_POINT('',(0.273180815962104,-0.292185286745036,0.45));
#38439=CARTESIAN_POINT('Ctrl Pts',(0.273180815962104,-0.292185286745036,
0.45));
#38440=CARTESIAN_POINT('Ctrl Pts',(0.269043642791963,-0.278239354461126,
0.463012481414242));
#38441=CARTESIAN_POINT('Ctrl Pts',(0.265165042944955,-0.265165042944955,
0.475));
#38442=CARTESIAN_POINT('',(0.273180815962104,-0.292185286745036,0.04));
#38443=CARTESIAN_POINT('',(0.273180815962104,-0.292185286745036,0.245));
#38444=CARTESIAN_POINT('Ctrl Pts',(0.265165042944955,-0.265165042944955,
0.015));
#38445=CARTESIAN_POINT('Ctrl Pts',(0.269043642791962,-0.278239354461121,
0.0269875185857534));
#38446=CARTESIAN_POINT('Ctrl Pts',(0.273180815962104,-0.292185286745036,
0.04));
#38447=CARTESIAN_POINT('Origin',(0.362222184858401,-0.0970571419134452,
0.5));
#38448=CARTESIAN_POINT('',(0.362222184858401,-0.0970571419134452,0.475));
#38449=CARTESIAN_POINT('',(0.389630288914294,-0.0904888830772255,0.45));
#38450=CARTESIAN_POINT('Ctrl Pts',(0.362222184858401,-0.0970571419134452,
0.475));
#38451=CARTESIAN_POINT('Ctrl Pts',(0.375484170691892,-0.0938789521539854,
0.463012481414249));
#38452=CARTESIAN_POINT('Ctrl Pts',(0.389630288914294,-0.0904888830772255,
0.45));
#38453=CARTESIAN_POINT('',(0.362222184858401,-0.0970571419134452,0.015));
#38454=CARTESIAN_POINT('',(0.362222184858401,-0.0970571419134452,0.5));
#38455=CARTESIAN_POINT('',(0.389630288914294,-0.0904888830772255,0.04));
#38456=CARTESIAN_POINT('Ctrl Pts',(0.389630288914294,-0.0904888830772256,
0.04));
#38457=CARTESIAN_POINT('Ctrl Pts',(0.375484170691905,-0.0938789521539823,
0.0269875185857627));
#38458=CARTESIAN_POINT('Ctrl Pts',(0.362222184858401,-0.0970571419134452,
0.015));
#38459=CARTESIAN_POINT('',(0.389630288914294,-0.0904888830772255,0.245));
#38460=CARTESIAN_POINT('Origin',(0.414762256080559,-0.146875018062859,0.5));
#38461=CARTESIAN_POINT('',(0.382674169822262,-0.11644947295219,0.45));
#38462=CARTESIAN_POINT('Ctrl Pts',(0.382674169822262,-0.11644947295219,
0.45));
#38463=CARTESIAN_POINT('Ctrl Pts',(0.372118306615106,-0.106440527899933,
0.463012481414245));
#38464=CARTESIAN_POINT('Ctrl Pts',(0.362222184858401,-0.0970571419134452,
0.475));
#38465=CARTESIAN_POINT('',(0.382674169822262,-0.11644947295219,0.04));
#38466=CARTESIAN_POINT('',(0.382674169822262,-0.11644947295219,0.245));
#38467=CARTESIAN_POINT('Ctrl Pts',(0.362222184858401,-0.0970571419134452,
0.015));
#38468=CARTESIAN_POINT('Ctrl Pts',(0.372118306615097,-0.106440527899925,
0.0269875185857436));
#38469=CARTESIAN_POINT('Ctrl Pts',(0.382674169822262,-0.11644947295219,
0.04));
#38470=CARTESIAN_POINT('Origin',(0.,0.,0.245));
#38471=CARTESIAN_POINT('Origin',(0.,0.,0.45));
#38472=CARTESIAN_POINT('Origin',(0.,0.,0.04));
#38473=CARTESIAN_POINT('Origin',(0.,0.,0.245));
#38474=CARTESIAN_POINT('Origin',(0.,0.,0.45));
#38475=CARTESIAN_POINT('Origin',(0.,0.,0.04));
#38476=CARTESIAN_POINT('Origin',(0.,0.,0.245));
#38477=CARTESIAN_POINT('Origin',(0.,0.,0.04));
#38478=CARTESIAN_POINT('Origin',(0.,0.,0.45));
#38479=CARTESIAN_POINT('Origin',(0.,0.,0.245));
#38480=CARTESIAN_POINT('Origin',(0.,0.,0.45));
#38481=CARTESIAN_POINT('Origin',(0.,0.,0.04));
#38482=CARTESIAN_POINT('Origin',(0.,0.,0.245));
#38483=CARTESIAN_POINT('Origin',(0.,0.,0.04));
#38484=CARTESIAN_POINT('Origin',(0.,0.,0.45));
#38485=CARTESIAN_POINT('Origin',(0.,0.,0.245));
#38486=CARTESIAN_POINT('Origin',(0.,0.,0.45));
#38487=CARTESIAN_POINT('Origin',(0.,0.,0.04));
#38488=CARTESIAN_POINT('Origin',(0.,0.,0.245));
#38489=CARTESIAN_POINT('Origin',(0.,0.,0.04));
#38490=CARTESIAN_POINT('Origin',(0.,0.,0.45));
#38491=CARTESIAN_POINT('Origin',(0.,0.,0.245));
#38492=CARTESIAN_POINT('Origin',(0.,0.,0.45));
#38493=CARTESIAN_POINT('Origin',(0.,0.,0.04));
#38494=CARTESIAN_POINT('Origin',(0.,0.,0.245));
#38495=CARTESIAN_POINT('Origin',(0.,0.,0.04));
#38496=CARTESIAN_POINT('Origin',(0.,0.,0.45));
#38497=CARTESIAN_POINT('Origin',(0.,0.,0.245));
#38498=CARTESIAN_POINT('Origin',(0.,0.,0.45));
#38499=CARTESIAN_POINT('Origin',(0.,0.,0.04));
#38500=CARTESIAN_POINT('Origin',(0.,0.,0.245));
#38501=CARTESIAN_POINT('Origin',(0.,0.,0.04));
#38502=CARTESIAN_POINT('Origin',(0.,0.,0.45));
#38503=CARTESIAN_POINT('Origin',(0.,0.,0.245));
#38504=CARTESIAN_POINT('Origin',(0.,0.,0.45));
#38505=CARTESIAN_POINT('Origin',(0.,0.,0.04));
#38506=CARTESIAN_POINT('Origin',(0.,0.,0.245));
#38507=CARTESIAN_POINT('Origin',(0.,0.,0.45));
#38508=CARTESIAN_POINT('Origin',(0.,0.,0.04));
#38509=CARTESIAN_POINT('Origin',(0.,0.,0.245));
#38510=CARTESIAN_POINT('Origin',(0.,0.,0.04));
#38511=CARTESIAN_POINT('Origin',(0.,0.,0.45));
#38512=CARTESIAN_POINT('Origin',(0.,0.,0.245));
#38513=CARTESIAN_POINT('Origin',(0.,0.,0.45));
#38514=CARTESIAN_POINT('Origin',(0.,0.,0.04));
#38515=CARTESIAN_POINT('Origin',(0.,0.,0.245));
#38516=CARTESIAN_POINT('Origin',(0.,0.,0.04));
#38517=CARTESIAN_POINT('Origin',(0.,0.,0.45));
#38518=CARTESIAN_POINT('Origin',(0.,0.,0.245));
#38519=CARTESIAN_POINT('Origin',(0.,0.,0.45));
#38520=CARTESIAN_POINT('Origin',(0.,0.,0.04));
#38521=CARTESIAN_POINT('Origin',(0.,0.,0.245));
#38522=CARTESIAN_POINT('Origin',(0.,0.,0.04));
#38523=CARTESIAN_POINT('Origin',(0.,0.,0.45));
#38524=CARTESIAN_POINT('Origin',(0.,0.,0.245));
#38525=CARTESIAN_POINT('Origin',(0.,0.,0.45));
#38526=CARTESIAN_POINT('Origin',(0.,0.,0.04));
#38527=CARTESIAN_POINT('Origin',(0.,0.,0.245));
#38528=CARTESIAN_POINT('Origin',(0.,0.,0.04));
#38529=CARTESIAN_POINT('Origin',(0.,0.,0.45));
#38530=CARTESIAN_POINT('Origin',(0.,0.,0.245));
#38531=CARTESIAN_POINT('Origin',(0.,0.,0.45));
#38532=CARTESIAN_POINT('Origin',(0.,0.,0.04));
#38533=CARTESIAN_POINT('Origin',(0.,0.,0.245));
#38534=CARTESIAN_POINT('Origin',(0.,0.,0.04));
#38535=CARTESIAN_POINT('Origin',(0.,0.,0.45));
#38536=CARTESIAN_POINT('Origin',(0.,0.,0.245));
#38537=CARTESIAN_POINT('Origin',(0.,0.,0.45));
#38538=CARTESIAN_POINT('Origin',(0.,0.,0.04));
#38539=CARTESIAN_POINT('Origin',(0.,0.,0.245));
#38540=CARTESIAN_POINT('Origin',(0.,0.,0.04));
#38541=CARTESIAN_POINT('Origin',(0.,0.,0.45));
#38542=CARTESIAN_POINT('Origin',(0.,0.,0.02));
#38543=CARTESIAN_POINT('',(-0.36,-4.40872847693047E-17,1.04083408558608E-17));
#38544=CARTESIAN_POINT('',(-0.38,-4.65365783675994E-17,0.02));
#38545=CARTESIAN_POINT('Origin',(0.,0.,0.));
#38546=CARTESIAN_POINT('Origin',(0.17,0.,-0.8));
#38547=CARTESIAN_POINT('',(-0.17,-2.0818995585505E-17,-0.8));
#38548=CARTESIAN_POINT('Origin',(0.,0.,-0.8));
#38549=CARTESIAN_POINT('Origin',(0.,0.,-0.785));
#38550=CARTESIAN_POINT('',(-0.185,-2.2655965784226E-17,-0.785));
#38551=CARTESIAN_POINT('Origin',(0.,0.,-0.385));
#38552=CARTESIAN_POINT('Origin',(0.,0.,0.));
#38553=CARTESIAN_POINT('Origin',(0.36,0.,0.));
#38554=CARTESIAN_POINT('Origin',(0.,0.,0.475));
#38555=CARTESIAN_POINT('',(-0.35,-4.28626379701574E-17,0.5));
#38556=CARTESIAN_POINT('Origin',(0.,0.,0.5));
#38557=CARTESIAN_POINT('',(-0.375,-4.59242549680257E-17,0.475));
#38558=CARTESIAN_POINT('Origin',(0.,0.,0.5));
#38594=UNCERTAINTY_MEASURE_WITH_UNIT(LENGTH_MEASURE(0.001),#38612,
'DISTANCE_ACCURACY_VALUE',
'Maximum model space distance between geometric entities at asserted c
onnectivities');
#38595=UNCERTAINTY_MEASURE_WITH_UNIT(LENGTH_MEASURE(0.001),#38612,
'DISTANCE_ACCURACY_VALUE',
'Maximum model space distance between geometric entities at asserted c
onnectivities');
#38610=(
GEOMETRIC_REPRESENTATION_CONTEXT(3)
GLOBAL_UNCERTAINTY_ASSIGNED_CONTEXT((#38594))
GLOBAL_UNIT_ASSIGNED_CONTEXT((#38612,#38614,#38615))
REPRESENTATION_CONTEXT('','3D')
);
#38611=(
GEOMETRIC_REPRESENTATION_CONTEXT(3)
GLOBAL_UNCERTAINTY_ASSIGNED_CONTEXT((#38595))
GLOBAL_UNIT_ASSIGNED_CONTEXT((#38612,#38614,#38615))
REPRESENTATION_CONTEXT('','3D')
);
#38612=(
LENGTH_UNIT()
NAMED_UNIT(*)
SI_UNIT(.CENTI.,.METRE.)
);
#38614=(
NAMED_UNIT(*)
PLANE_ANGLE_UNIT()
SI_UNIT($,.RADIAN.)
);
#38615=(
NAMED_UNIT(*)
SI_UNIT($,.STERADIAN.)
SOLID_ANGLE_UNIT()
);
#38630=SHAPE_DEFINITION_REPRESENTATION(#38645,#38681);
#38645=PRODUCT_DEFINITION_SHAPE('',$,#38697);
#38681=SHAPE_REPRESENTATION('',(#17623),#38610);
#38682=PRODUCT_DEFINITION_CONTEXT('part definition',#38729,'design');
#38697=PRODUCT_DEFINITION('2026-10-19-02-32-05-072',
'12_Brass_Knurled_Thumb_Lock_Screw_M4x8',#38712,#38682);
#38712=PRODUCT_DEFINITION_FORMATION('',$,#38745);
#38729=APPLICATION_CONTEXT(
'Core Data for Automotive Mechanical Design Process');
#38730=PRODUCT_CONTEXT('part definition',#38729,'mechanical');
#38745=PRODUCT('2026-10-19-02-32-05-072',
'12_Brass_Knurled_Thumb_Lock_Screw_M4x8',$,(#38730));
#38879=COLOUR_RGB('Black',0.12,0.14,0.17);
#38880=FILL_AREA_STYLE_COLOUR('',#38879);
#38881=FILL_AREA_STYLE('',(#38880));
#38882=SURFACE_STYLE_FILL_AREA(#38881);
#38883=SURFACE_SIDE_STYLE('',(#38882));
#38884=SURFACE_STYLE_USAGE(.BOTH.,#38883);
#38885=PRESENTATION_STYLE_ASSIGNMENT((#38884));
ENDSEC;
END-ISO-10303-21;
